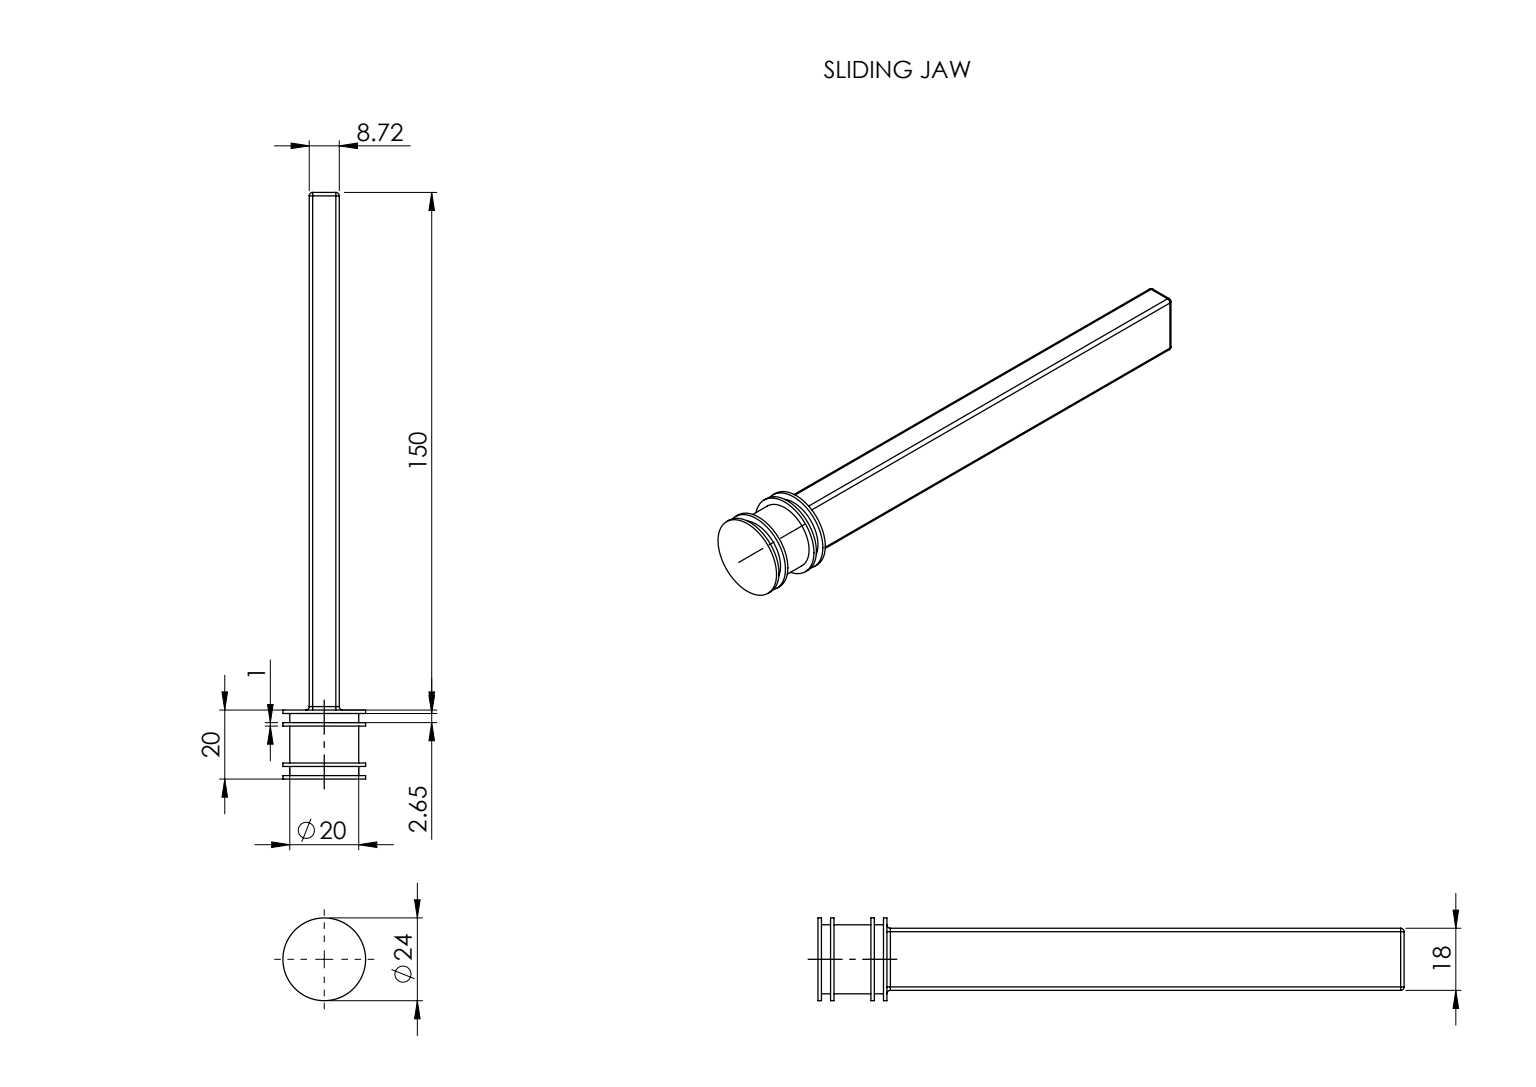
ISO-10303-21;
HEADER;
FILE_DESCRIPTION (('STEP AP214'),
    '1' );
FILE_NAME ('sliding jaw.step',
    '2026-09-29T11:11:29',
    ( '' ),
    ( '' ),
    'SwSTEP 2.0',
    'SolidWorks 2026',
    '' );
FILE_SCHEMA (( 'AUTOMOTIVE_DESIGN' ));
ENDSEC;

DATA;
#4=ORIENTED_EDGE ( 'NONE', *, *, #636, .F. ) ;
#16=DIRECTION ( 'NONE',  ( 0.000000000000000000, 0.000000000000000000, 1.000000000000000000 ) ) ;
#25=DIRECTION ( 'NONE',  ( 1.000000000000000000, 0.000000000000000000, 0.000000000000000000 ) ) ;
#52=CIRCLE ( 'NONE', #6511, 10.00000000000000178 ) ;
#59=CARTESIAN_POINT ( 'NONE',  ( -33.35889894354067309, -7.999999999999996447, -25.00000000000000000 ) ) ;
#82=CARTESIAN_POINT ( 'NONE',  ( -30.00000000000002842, 0.000000000000000000, -44.00000000000000000 ) ) ;
#86=AXIS2_PLACEMENT_3D ( 'NONE', #4207, #8514, #2479 ) ;
#93=SHAPE_DEFINITION_REPRESENTATION ( #6343, #4062 ) ;
#96=CIRCLE ( 'NONE', #1362, 10.00000000000000178 ) ;
#112=VERTEX_POINT ( 'NONE', #3443 ) ;
#118=CARTESIAN_POINT ( 'NONE',  ( -26.64110105645932336, -7.999999999999996447, -23.99999999999999289 ) ) ;
#123=ORIENTED_EDGE ( 'NONE', *, *, #7045, .T. ) ;
#128=CARTESIAN_POINT ( 'NONE',  ( -30.00000000000002842, 0.000000000000000000, -45.00000000000000000 ) ) ;
#157=CIRCLE ( 'NONE', #7186, 11.99999999999979217 ) ;
#159=EDGE_LOOP ( 'NONE', ( #5400, #1966 ) ) ;
#162=CARTESIAN_POINT ( 'NONE',  ( -30.00000000000002842, 0.000000000000000000, -28.65000000000000213 ) ) ;
#164=CARTESIAN_POINT ( 'NONE',  ( -30.00000000000002487, 0.000000000000000000, -25.00000000000000000 ) ) ;
#165=DIRECTION ( 'NONE',  ( -0.000000000000000000, -0.000000000000000000, -1.000000000000000000 ) ) ;
#169=EDGE_LOOP ( 'NONE', ( #3481, #7886, #4, #4040 ) ) ;
#183=CARTESIAN_POINT ( 'NONE',  ( -30.00000000000002842, 10.00000000000000178, -24.00000000000000000 ) ) ;
#194=ORIENTED_EDGE ( 'NONE', *, *, #7448, .F. ) ;
#195=CARTESIAN_POINT ( 'NONE',  ( -33.35889894354067309, -9.999999999999998224, -25.00000000000000000 ) ) ;
#203=FACE_BOUND ( 'NONE', #7034, .T. ) ;
#206=DIRECTION ( 'NONE',  ( -1.000000000000000000, 0.000000000000000000, 0.000000000000000000 ) ) ;
#220=AXIS2_PLACEMENT_3D ( 'NONE', #5235, #7767, #7308 ) ;
#222=CYLINDRICAL_SURFACE ( 'NONE', #8532, 1.000000000000000888 ) ;
#224=LINE ( 'NONE', #3711, #2134 ) ;
#229=CYLINDRICAL_SURFACE ( 'NONE', #3390, 10.00000000000000178 ) ;
#244=PLANE ( 'NONE',  #7417 ) ;
#265=FACE_OUTER_BOUND ( 'NONE', #169, .T. ) ;
#276=CARTESIAN_POINT ( 'NONE',  ( -30.00000000000002487, 0.000000000000000000, -40.35000000000000142 ) ) ;
#280=DIRECTION ( 'NONE',  ( 1.000000000000000000, 0.000000000000000000, 0.000000000000000000 ) ) ;
#300=DIRECTION ( 'NONE',  ( 0.000000000000000000, 0.000000000000000000, 1.000000000000000000 ) ) ;
#303=DIRECTION ( 'NONE',  ( -0.000000000000000000, -0.000000000000000000, -1.000000000000000000 ) ) ;
#315=AXIS2_PLACEMENT_3D ( 'NONE', #2642, #5313, #2599 ) ;
#319=CARTESIAN_POINT ( 'NONE',  ( -26.64110105645932336, -7.999999999999996447, 125.0000000000000000 ) ) ;
#331=SPHERICAL_SURFACE ( 'NONE', #3585, 1.000000000000000000 ) ;
#340=CARTESIAN_POINT ( 'NONE',  ( -26.64110105645932336, 8.000000000000000000, 124.0000000000000000 ) ) ;
#342=DIRECTION ( 'NONE',  ( -1.000000000000000000, 0.000000000000000000, 0.000000000000000000 ) ) ;
#360=EDGE_LOOP ( 'NONE', ( #4155, #3028, #6612 ) ) ;
#381=CARTESIAN_POINT ( 'NONE',  ( -33.35889894354067309, -7.999999999999996447, 124.0000000000000000 ) ) ;
#387=EDGE_LOOP ( 'NONE', ( #8592, #8016, #455, #3412 ) ) ;
#390=PLANE ( 'NONE',  #4662 ) ;
#391=DIRECTION ( 'NONE',  ( 0.000000000000000000, 0.000000000000000000, -1.000000000000000000 ) ) ;
#396=DIRECTION ( 'NONE',  ( 0.000000000000000000, 0.000000000000000000, -1.000000000000000000 ) ) ;
#408=CIRCLE ( 'NONE', #1969, 1.000000000000000888 ) ;
#419=FACE_OUTER_BOUND ( 'NONE', #3879, .T. ) ;
#431=LINE ( 'NONE', #3098, #1438 ) ;
#441=EDGE_CURVE ( 'NONE', #598, #864, #8558, .T. ) ;
#450=ORIENTED_EDGE ( 'NONE', *, *, #3020, .T. ) ;
#455=ORIENTED_EDGE ( 'NONE', *, *, #8086, .F. ) ;
#460=CARTESIAN_POINT ( 'NONE',  ( -30.00000000000002487, 0.000000000000000000, -29.65000000000000213 ) ) ;
#463=ORIENTED_EDGE ( 'NONE', *, *, #2478, .F. ) ;
#466=AXIS2_PLACEMENT_3D ( 'NONE', #6133, #6787, #2038 ) ;
#469=CARTESIAN_POINT ( 'NONE',  ( -26.64110105645932336, 8.000000000000000000, -23.99999999999999289 ) ) ;
#471=CARTESIAN_POINT ( 'NONE',  ( -33.35889894354067309, 8.000000000000000000, 125.0000000000000000 ) ) ;
#477=ORIENTED_EDGE ( 'NONE', *, *, #3290, .F. ) ;
#487=CARTESIAN_POINT ( 'NONE',  ( -18.00000000000023093, 1.469576158976798506E-15, -45.00000000000000000 ) ) ;
#489=TOROIDAL_SURFACE ( 'NONE', #7690, 2.000000000000000000, 1.000000000000000000 ) ;
#506=AXIS2_PLACEMENT_3D ( 'NONE', #7866, #2374, #8526 ) ;
#508=ADVANCED_FACE ( 'NONE', ( #3062, #1146 ), #5739, .F. ) ;
#511=DIRECTION ( 'NONE',  ( 0.000000000000000000, 0.000000000000000000, 1.000000000000000000 ) ) ;
#520=DIRECTION ( 'NONE',  ( 0.000000000000000000, 0.000000000000000000, 1.000000000000000000 ) ) ;
#527=CLOSED_SHELL ( 'NONE', ( #5613, #7239, #5879, #6349, #2268, #2193, #5062, #3908, #2590, #5355, #6240, #6891, #7681, #6961, #3590, #7937, #508, #6501, #1125, #2411, #1851, #6598, #8377, #3918, #1178, #796, #1378, #5792, #2216, #3557, #4936, #1316, #7178, #7893, #8060, #1449, #7304, #1330, #3411, #2383, #6115, #1171, #7572, #8073, #5454, #4555, #3146 ) ) ;
#536=( NAMED_UNIT ( * ) SI_UNIT ( $, .STERADIAN. ) SOLID_ANGLE_UNIT ( ) );
#537=ORIENTED_EDGE ( 'NONE', *, *, #6250, .F. ) ;
#538=DIRECTION ( 'NONE',  ( 0.000000000000000000, 0.000000000000000000, -1.000000000000000000 ) ) ;
#563=CARTESIAN_POINT ( 'NONE',  ( -42.00000000000002132, 0.000000000000000000, -29.65000000000000213 ) ) ;
#572=PLANE ( 'NONE',  #1496 ) ;
#580=VERTEX_POINT ( 'NONE', #7145 ) ;
#586=ORIENTED_EDGE ( 'NONE', *, *, #2638, .T. ) ;
#590=( LENGTH_UNIT ( ) NAMED_UNIT ( * ) SI_UNIT ( .MILLI., .METRE. ) );
#595=EDGE_LOOP ( 'NONE', ( #4745, #2458, #2730, #1335 ) ) ;
#598=VERTEX_POINT ( 'NONE', #8559 ) ;
#615=CARTESIAN_POINT ( 'NONE',  ( -26.64110105645932336, 9.000000000000001776, 125.0000000000000000 ) ) ;
#618=LINE ( 'NONE', #2581, #6843 ) ;
#627=AXIS2_PLACEMENT_3D ( 'NONE', #1489, #300, #3700 ) ;
#636=EDGE_CURVE ( 'NONE', #5681, #7609, #5596, .T. ) ;
#644=DIRECTION ( 'NONE',  ( 1.000000000000000000, 0.000000000000000000, 0.000000000000000000 ) ) ;
#653=AXIS2_PLACEMENT_3D ( 'NONE', #4860, #1588, #6305 ) ;
#658=CARTESIAN_POINT ( 'NONE',  ( -17.99999999999998579, 1.469576158976828483E-15, -29.65000000000000213 ) ) ;
#659=DIRECTION ( 'NONE',  ( -0.000000000000000000, -0.000000000000000000, -1.000000000000000000 ) ) ;
#661=ORIENTED_EDGE ( 'NONE', *, *, #5691, .T. ) ;
#673=ORIENTED_EDGE ( 'NONE', *, *, #4128, .F. ) ;
#697=DIRECTION ( 'NONE',  ( -1.000000000000000000, 0.000000000000000000, 0.000000000000000000 ) ) ;
#706=AXIS2_PLACEMENT_3D ( 'NONE', #5991, #697, #8325 ) ;
#714=CARTESIAN_POINT ( 'NONE',  ( -40.00000000000002842, 1.224646799147353059E-15, -40.35000000000000142 ) ) ;
#725=ORIENTED_EDGE ( 'NONE', *, *, #7163, .T. ) ;
#731=DIRECTION ( 'NONE',  ( 0.000000000000000000, -1.000000000000000000, 0.000000000000000000 ) ) ;
#733=ORIENTED_EDGE ( 'NONE', *, *, #8138, .T. ) ;
#771=EDGE_CURVE ( 'NONE', #772, #7794, #6358, .T. ) ;
#772=VERTEX_POINT ( 'NONE', #3873 ) ;
#774=CARTESIAN_POINT ( 'NONE',  ( -26.64110105645932336, -9.999999999999998224, -24.00000000000000000 ) ) ;
#776=DIRECTION ( 'NONE',  ( -1.000000000000000000, 0.000000000000000000, 0.000000000000000000 ) ) ;
#796=ADVANCED_FACE ( 'NONE', ( #3827 ), #6507, .T. ) ;
#806=DIRECTION ( 'NONE',  ( 1.000000000000000000, 0.000000000000000000, -0.000000000000000000 ) ) ;
#812=ORIENTED_EDGE ( 'NONE', *, *, #2573, .F. ) ;
#818=EDGE_CURVE ( 'NONE', #7794, #1195, #3435, .T. ) ;
#822=CARTESIAN_POINT ( 'NONE',  ( -30.00000000000002842, 0.000000000000000000, -40.35000000000000142 ) ) ;
#824=ORIENTED_EDGE ( 'NONE', *, *, #8649, .T. ) ;
#830=CARTESIAN_POINT ( 'NONE',  ( -33.35889894354067309, -7.999999999999996447, -23.99999999999999289 ) ) ;
#849=CIRCLE ( 'NONE', #6478, 10.00000000000000178 ) ;
#852=PLANE ( 'NONE',  #1788 ) ;
#853=ORIENTED_EDGE ( 'NONE', *, *, #886, .F. ) ;
#859=CARTESIAN_POINT ( 'NONE',  ( -20.00000000000002487, 0.000000000000000000, -41.34999999999999432 ) ) ;
#860=DIRECTION ( 'NONE',  ( 0.000000000000000000, 0.000000000000000000, 1.000000000000000000 ) ) ;
#862=CARTESIAN_POINT ( 'NONE',  ( -30.00000000000002487, 0.000000000000000000, -29.65000000000000213 ) ) ;
#864=VERTEX_POINT ( 'NONE', #1218 ) ;
#881=AXIS2_PLACEMENT_3D ( 'NONE', #1764, #2549, #8503 ) ;
#886=EDGE_CURVE ( 'NONE', #2202, #3619, #5942, .T. ) ;
#888=AXIS2_PLACEMENT_3D ( 'NONE', #1840, #2501, #538 ) ;
#893=EDGE_CURVE ( 'NONE', #4571, #5715, #1301, .T. ) ;
#903=VECTOR ( 'NONE', #7606, 1000.000000000000000 ) ;
#909=LINE ( 'NONE', #6766, #903 ) ;
#931=CARTESIAN_POINT ( 'NONE',  ( -40.00000000000002842, 1.224646799147353059E-15, -26.00000000000000355 ) ) ;
#932=TOROIDAL_SURFACE ( 'NONE', #1494, 2.000000000000000000, 1.000000000000000000 ) ;
#946=AXIS2_PLACEMENT_3D ( 'NONE', #774, #5439, #860 ) ;
#950=CARTESIAN_POINT ( 'NONE',  ( -26.64110105645932336, -8.999999999999998224, -24.00000000000000000 ) ) ;
#952=DIRECTION ( 'NONE',  ( 0.000000000000000000, 0.000000000000000000, 1.000000000000000000 ) ) ;
#955=ORIENTED_EDGE ( 'NONE', *, *, #6438, .T. ) ;
#959=EDGE_LOOP ( 'NONE', ( #4655, #2762 ) ) ;
#964=CARTESIAN_POINT ( 'NONE',  ( -34.35889894354067309, -8.999999999999998224, -24.00000000000000000 ) ) ;
#973=DIRECTION ( 'NONE',  ( 0.000000000000000000, 0.000000000000000000, 1.000000000000000000 ) ) ;
#989=CARTESIAN_POINT ( 'NONE',  ( -26.64110105645932336, 9.000000000000001776, -24.00000000000000000 ) ) ;
#998=CIRCLE ( 'NONE', #4381, 1.000000000000000888 ) ;
#999=VERTEX_POINT ( 'NONE', #7967 ) ;
#1007=EDGE_CURVE ( 'NONE', #4525, #7472, #6705, .T. ) ;
#1009=VERTEX_POINT ( 'NONE', #4000 ) ;
#1012=ORIENTED_EDGE ( 'NONE', *, *, #6438, .F. ) ;
#1019=DIRECTION ( 'NONE',  ( -0.000000000000000000, -0.000000000000000000, -1.000000000000000000 ) ) ;
#1021=CIRCLE ( 'NONE', #5949, 1.000000000000000888 ) ;
#1039=CARTESIAN_POINT ( 'NONE',  ( -35.35889894354067309, 0.000000000000000000, -24.00000000000000000 ) ) ;
#1044=CIRCLE ( 'NONE', #6810, 10.00000000000000178 ) ;
#1046=VERTEX_POINT ( 'NONE', #950 ) ;
#1059=DIRECTION ( 'NONE',  ( 0.000000000000000000, 0.000000000000000000, -1.000000000000000000 ) ) ;
#1065=CARTESIAN_POINT ( 'NONE',  ( -33.35889894354067309, 10.00000000000000178, -25.00000000000000000 ) ) ;
#1072=VERTEX_POINT ( 'NONE', #3758 ) ;
#1083=EDGE_LOOP ( 'NONE', ( #3654, #4068, #5069, #1575 ) ) ;
#1092=CARTESIAN_POINT ( 'NONE',  ( -25.64110105645932336, 8.000000000000000000, 125.0000000000000000 ) ) ;
#1094=FACE_OUTER_BOUND ( 'NONE', #2864, .T. ) ;
#1112=ORIENTED_EDGE ( 'NONE', *, *, #3664, .T. ) ;
#1117=CARTESIAN_POINT ( 'NONE',  ( -42.00000000000002132, 0.000000000000000000, -28.65000000000000213 ) ) ;
#1125=ADVANCED_FACE ( 'NONE', ( #203, #4882 ), #244, .F. ) ;
#1146=FACE_OUTER_BOUND ( 'NONE', #3517, .T. ) ;
#1148=EDGE_CURVE ( 'NONE', #1263, #1046, #2502, .T. ) ;
#1157=EDGE_CURVE ( 'NONE', #4571, #3127, #4461, .T. ) ;
#1164=DIRECTION ( 'NONE',  ( -1.000000000000000000, 0.000000000000000000, 0.000000000000000000 ) ) ;
#1171=ADVANCED_FACE ( 'NONE', ( #4922 ), #8239, .T. ) ;
#1172=CIRCLE ( 'NONE', #6516, 10.00000000000000178 ) ;
#1177=CARTESIAN_POINT ( 'NONE',  ( -42.00000000000006395, 0.000000000000000000, -29.65000000000000213 ) ) ;
#1178=ADVANCED_FACE ( 'NONE', ( #5574, #8282 ), #2243, .F. ) ;
#1182=VECTOR ( 'NONE', #7954, 1000.000000000000000 ) ;
#1183=ORIENTED_EDGE ( 'NONE', *, *, #2611, .F. ) ;
#1189=EDGE_CURVE ( 'NONE', #5443, #1675, #4966, .T. ) ;
#1192=DIRECTION ( 'NONE',  ( -0.000000000000000000, 1.000000000000000000, 0.000000000000000000 ) ) ;
#1195=VERTEX_POINT ( 'NONE', #2111 ) ;
#1208=AXIS2_PLACEMENT_3D ( 'NONE', #2158, #8155, #3438 ) ;
#1215=ORIENTED_EDGE ( 'NONE', *, *, #8346, .F. ) ;
#1218=CARTESIAN_POINT ( 'NONE',  ( -24.64110105645932336, 8.000000000000000000, -25.00000000000000000 ) ) ;
#1219=FACE_OUTER_BOUND ( 'NONE', #2950, .T. ) ;
#1226=CYLINDRICAL_SURFACE ( 'NONE', #220, 12.00000000000000000 ) ;
#1235=CARTESIAN_POINT ( 'NONE',  ( -24.64110105645932336, -8.999999999999998224, -25.00000000000000000 ) ) ;
#1239=DIRECTION ( 'NONE',  ( 0.000000000000000000, 1.000000000000000000, -0.000000000000000000 ) ) ;
#1243=DIRECTION ( 'NONE',  ( -0.000000000000000000, -0.000000000000000000, -1.000000000000000000 ) ) ;
#1254=ORIENTED_EDGE ( 'NONE', *, *, #636, .T. ) ;
#1263=VERTEX_POINT ( 'NONE', #6917 ) ;
#1265=EDGE_CURVE ( 'NONE', #2617, #8337, #8133, .T. ) ;
#1275=DIRECTION ( 'NONE',  ( -1.000000000000000000, 0.000000000000000000, 0.000000000000000000 ) ) ;
#1279=CARTESIAN_POINT ( 'NONE',  ( -24.64110105645932336, 0.000000000000000000, -24.00000000000000000 ) ) ;
#1287=LINE ( 'NONE', #5256, #1182 ) ;
#1300=( NAMED_UNIT ( * ) PLANE_ANGLE_UNIT ( ) SI_UNIT ( $, .RADIAN. ) );
#1301=LINE ( 'NONE', #5396, #2999 ) ;
#1316=ADVANCED_FACE ( 'NONE', ( #2172 ), #222, .F. ) ;
#1321=CARTESIAN_POINT ( 'NONE',  ( -34.35889894354067309, 8.000000000000000000, 124.0000000000000000 ) ) ;
#1327=CARTESIAN_POINT ( 'NONE',  ( -26.64110105645932336, -7.999999999999996447, 124.0000000000000000 ) ) ;
#1330=ADVANCED_FACE ( 'NONE', ( #265 ), #489, .F. ) ;
#1332=CYLINDRICAL_SURFACE ( 'NONE', #3852, 1.000000000000000888 ) ;
#1334=( NAMED_UNIT ( * ) PLANE_ANGLE_UNIT ( ) SI_UNIT ( $, .RADIAN. ) );
#1335=ORIENTED_EDGE ( 'NONE', *, *, #5477, .T. ) ;
#1345=DIRECTION ( 'NONE',  ( -1.000000000000000000, 0.000000000000000000, 0.000000000000000000 ) ) ;
#1348=CARTESIAN_POINT ( 'NONE',  ( -30.00000000000002842, 0.000000000000000000, -45.00000000000000000 ) ) ;
#1362=AXIS2_PLACEMENT_3D ( 'NONE', #5707, #8409, #1701 ) ;
#1378=ADVANCED_FACE ( 'NONE', ( #6728 ), #5228, .F. ) ;
#1388=ORIENTED_EDGE ( 'NONE', *, *, #8346, .T. ) ;
#1389=EDGE_LOOP ( 'NONE', ( #2321, #2903 ) ) ;
#1391=CARTESIAN_POINT ( 'NONE',  ( -25.64110105645932336, 8.000000000000000000, 124.0000000000000000 ) ) ;
#1394=DIRECTION ( 'NONE',  ( 0.000000000000000000, 0.000000000000000000, -1.000000000000000000 ) ) ;
#1395=CARTESIAN_POINT ( 'NONE',  ( -35.35889894354067309, 8.000000000000000000, -24.00000000000000000 ) ) ;
#1427=EDGE_LOOP ( 'NONE', ( #3891, #3996 ) ) ;
#1438=VECTOR ( 'NONE', #5779, 1000.000000000000000 ) ;
#1443=ORIENTED_EDGE ( 'NONE', *, *, #6341, .T. ) ;
#1449=ADVANCED_FACE ( 'NONE', ( #8285 ), #2862, .T. ) ;
#1464=EDGE_CURVE ( 'NONE', #8429, #5042, #3565, .T. ) ;
#1472=ORIENTED_EDGE ( 'NONE', *, *, #6300, .T. ) ;
#1481=CARTESIAN_POINT ( 'NONE',  ( -34.35889894354067309, -7.999999999999996447, 125.0000000000000000 ) ) ;
#1486=EDGE_LOOP ( 'NONE', ( #3350, #2470 ) ) ;
#1489=CARTESIAN_POINT ( 'NONE',  ( -30.00000000000002842, 0.000000000000000000, -45.00000000000000000 ) ) ;
#1494=AXIS2_PLACEMENT_3D ( 'NONE', #7551, #1514, #280 ) ;
#1496=AXIS2_PLACEMENT_3D ( 'NONE', #3239, #2709, #6749 ) ;
#1503=AXIS2_PLACEMENT_3D ( 'NONE', #3408, #7897, #1275 ) ;
#1508=AXIS2_PLACEMENT_3D ( 'NONE', #5913, #2660, #8687 ) ;
#1514=DIRECTION ( 'NONE',  ( 0.000000000000000000, 0.000000000000000000, 1.000000000000000000 ) ) ;
#1519=ORIENTED_EDGE ( 'NONE', *, *, #1781, .F. ) ;
#1522=DIRECTION ( 'NONE',  ( -1.000000000000000000, 0.000000000000000000, 0.000000000000000000 ) ) ;
#1537=ORIENTED_EDGE ( 'NONE', *, *, #4588, .T. ) ;
#1545=CARTESIAN_POINT ( 'NONE',  ( -30.00000000000002842, 0.000000000000000000, -41.34999999999999432 ) ) ;
#1554=VECTOR ( 'NONE', #2289, 1000.000000000000000 ) ;
#1558=ORIENTED_EDGE ( 'NONE', *, *, #7155, .F. ) ;
#1567=LINE ( 'NONE', #7478, #7656 ) ;
#1575=ORIENTED_EDGE ( 'NONE', *, *, #6921, .F. ) ;
#1581=DIRECTION ( 'NONE',  ( 0.000000000000000000, 0.000000000000000000, 1.000000000000000000 ) ) ;
#1583=ORIENTED_EDGE ( 'NONE', *, *, #2646, .F. ) ;
#1587=AXIS2_PLACEMENT_3D ( 'NONE', #2835, #3455, #8171 ) ;
#1588=DIRECTION ( 'NONE',  ( 0.000000000000000000, -0.000000000000000000, 1.000000000000000000 ) ) ;
#1590=CARTESIAN_POINT ( 'NONE',  ( -33.35889894354067309, -9.999999999999998224, -24.00000000000000000 ) ) ;
#1604=ORIENTED_EDGE ( 'NONE', *, *, #8180, .F. ) ;
#1608=AXIS2_PLACEMENT_3D ( 'NONE', #2572, #5245, #8717 ) ;
#1609=EDGE_CURVE ( 'NONE', #3466, #3121, #6430, .T. ) ;
#1612=CARTESIAN_POINT ( 'NONE',  ( -30.00000000000023093, 0.000000000000000000, -44.00000000000000000 ) ) ;
#1616=DIRECTION ( 'NONE',  ( 0.000000000000000000, 0.000000000000000000, 1.000000000000000000 ) ) ;
#1642=EDGE_CURVE ( 'NONE', #3619, #6952, #5026, .T. ) ;
#1647=CIRCLE ( 'NONE', #6298, 1.000000000000000888 ) ;
#1654=VECTOR ( 'NONE', #2362, 1000.000000000000000 ) ;
#1660=CARTESIAN_POINT ( 'NONE',  ( -26.64110105645932336, -7.999999999999996447, 124.0000000000000000 ) ) ;
#1663=VERTEX_POINT ( 'NONE', #859 ) ;
#1675=VERTEX_POINT ( 'NONE', #6365 ) ;
#1679=DIRECTION ( 'NONE',  ( 0.000000000000000000, 0.000000000000000000, 1.000000000000000000 ) ) ;
#1681=LINE ( 'NONE', #6437, #4511 ) ;
#1690=CARTESIAN_POINT ( 'NONE',  ( -41.99999999999981526, 0.000000000000000000, -44.00000000000000000 ) ) ;
#1694=ORIENTED_EDGE ( 'NONE', *, *, #3020, .F. ) ;
#1701=DIRECTION ( 'NONE',  ( 1.000000000000000000, 0.000000000000000000, 0.000000000000000000 ) ) ;
#1707=DIRECTION ( 'NONE',  ( 0.000000000000000000, 0.000000000000000000, 1.000000000000000000 ) ) ;
#1719=DIRECTION ( 'NONE',  ( -1.000000000000000000, 0.000000000000000000, 0.000000000000000000 ) ) ;
#1721=ORIENTED_EDGE ( 'NONE', *, *, #1642, .T. ) ;
#1723=EDGE_CURVE ( 'NONE', #1046, #5443, #2412, .T. ) ;
#1731=FACE_BOUND ( 'NONE', #6833, .T. ) ;
#1732=DIRECTION ( 'NONE',  ( -1.000000000000000000, 0.000000000000000000, 0.000000000000000000 ) ) ;
#1735=VECTOR ( 'NONE', #3213, 1000.000000000000000 ) ;
#1744=VECTOR ( 'NONE', #7293, 1000.000000000000000 ) ;
#1757=ORIENTED_EDGE ( 'NONE', *, *, #818, .F. ) ;
#1764=CARTESIAN_POINT ( 'NONE',  ( -30.00000000000002487, 0.000000000000000000, -41.35000000000000142 ) ) ;
#1775=DIRECTION ( 'NONE',  ( 1.000000000000000000, 0.000000000000000000, -0.000000000000000000 ) ) ;
#1776=AXIS2_PLACEMENT_3D ( 'NONE', #4486, #5186, #6424 ) ;
#1779=CARTESIAN_POINT ( 'NONE',  ( -30.00000000000002487, 0.000000000000000000, -28.65000000000000213 ) ) ;
#1781=EDGE_CURVE ( 'NONE', #5443, #3221, #5287, .T. ) ;
#1782=DIRECTION ( 'NONE',  ( 1.000000000000000000, 0.000000000000000000, 0.000000000000000000 ) ) ;
#1788=AXIS2_PLACEMENT_3D ( 'NONE', #4252, #2234, #6318 ) ;
#1793=FACE_OUTER_BOUND ( 'NONE', #1083, .T. ) ;
#1801=ORIENTED_EDGE ( 'NONE', *, *, #8649, .F. ) ;
#1805=CARTESIAN_POINT ( 'NONE',  ( -40.00000000000002842, 1.224646799147353256E-15, -45.00000000000000000 ) ) ;
#1822=EDGE_CURVE ( 'NONE', #3764, #5405, #618, .T. ) ;
#1830=CARTESIAN_POINT ( 'NONE',  ( -34.35889894354067309, 9.000000000000001776, 125.0000000000000000 ) ) ;
#1840=CARTESIAN_POINT ( 'NONE',  ( -33.35889894354067309, -8.999999999999998224, 124.0000000000000000 ) ) ;
#1848=LINE ( 'NONE', #3787, #7361 ) ;
#1851=ADVANCED_FACE ( 'NONE', ( #7906, #1872 ), #572, .F. ) ;
#1861=DIRECTION ( 'NONE',  ( -0.000000000000000000, -1.000000000000000000, -0.000000000000000000 ) ) ;
#1872=FACE_OUTER_BOUND ( 'NONE', #3259, .T. ) ;
#1877=DIRECTION ( 'NONE',  ( 0.000000000000000000, 0.000000000000000000, 1.000000000000000000 ) ) ;
#1878=CIRCLE ( 'NONE', #881, 11.99999999999983302 ) ;
#1893=AXIS2_PLACEMENT_3D ( 'NONE', #164, #2861, #5536 ) ;
#1896=ORIENTED_EDGE ( 'NONE', *, *, #8180, .T. ) ;
#1901=CARTESIAN_POINT ( 'NONE',  ( -20.00000000000002487, 0.000000000000000000, -40.35000000000000142 ) ) ;
#1905=DIRECTION ( 'NONE',  ( -0.000000000000000000, -0.000000000000000000, -1.000000000000000000 ) ) ;
#1925=VERTEX_POINT ( 'NONE', #2532 ) ;
#1926=AXIS2_PLACEMENT_3D ( 'NONE', #4885, #165, #206 ) ;
#1930=CARTESIAN_POINT ( 'NONE',  ( -30.00000000000002487, 0.000000000000000000, -45.00000000000000000 ) ) ;
#1934=ORIENTED_EDGE ( 'NONE', *, *, #3311, .T. ) ;
#1935=AXIS2_PLACEMENT_3D ( 'NONE', #8305, #6923, #2178 ) ;
#1961=DIRECTION ( 'NONE',  ( -1.000000000000000000, -0.000000000000000000, -0.000000000000000000 ) ) ;
#1965=ORIENTED_EDGE ( 'NONE', *, *, #7880, .T. ) ;
#1966=ORIENTED_EDGE ( 'NONE', *, *, #7163, .F. ) ;
#1969=AXIS2_PLACEMENT_3D ( 'NONE', #6964, #3095, #5117 ) ;
#1978=AXIS2_PLACEMENT_3D ( 'NONE', #4643, #7423, #7331 ) ;
#1982=CIRCLE ( 'NONE', #5347, 1.000000000000000888 ) ;
#1987=( GEOMETRIC_REPRESENTATION_CONTEXT ( 3 ) GLOBAL_UNCERTAINTY_ASSIGNED_CONTEXT ( ( #3854 ) ) GLOBAL_UNIT_ASSIGNED_CONTEXT ( ( #8044, #1334, #536 ) ) REPRESENTATION_CONTEXT ( 'NONE', 'WORKASPACE' ) );
#1991=FACE_OUTER_BOUND ( 'NONE', #3804, .T. ) ;
#1994=ORIENTED_EDGE ( 'NONE', *, *, #7332, .T. ) ;
#2003=PLANE ( 'NONE',  #4144 ) ;
#2005=( NAMED_UNIT ( * ) PLANE_ANGLE_UNIT ( ) SI_UNIT ( $, .RADIAN. ) );
#2018=DIRECTION ( 'NONE',  ( 1.000000000000000000, -0.000000000000000000, -0.000000000000000000 ) ) ;
#2034=CIRCLE ( 'NONE', #1893, 12.00000000000004263 ) ;
#2038=DIRECTION ( 'NONE',  ( 1.000000000000000000, 0.000000000000000000, 0.000000000000000000 ) ) ;
#2041=LINE ( 'NONE', #615, #2787 ) ;
#2053=DIRECTION ( 'NONE',  ( 1.000000000000000000, 0.000000000000000000, 0.000000000000000000 ) ) ;
#2085=DIRECTION ( 'NONE',  ( -1.000000000000000000, -0.000000000000000000, 0.000000000000000000 ) ) ;
#2101=DIRECTION ( 'NONE',  ( 0.000000000000000000, 0.000000000000000000, 1.000000000000000000 ) ) ;
#2110=FILL_AREA_STYLE_COLOUR ( '', #8071 ) ;
#2111=CARTESIAN_POINT ( 'NONE',  ( -26.64110105645932336, -7.999999999999996447, 125.0000000000000000 ) ) ;
#2134=VECTOR ( 'NONE', #1059, 1000.000000000000000 ) ;
#2141=FACE_BOUND ( 'NONE', #3876, .T. ) ;
#2145=ORIENTED_EDGE ( 'NONE', *, *, #7045, .F. ) ;
#2150=VERTEX_POINT ( 'NONE', #3923 ) ;
#2154=VECTOR ( 'NONE', #1019, 1000.000000000000000 ) ;
#2155=DIRECTION ( 'NONE',  ( 1.000000000000000000, 0.000000000000000000, -0.000000000000000000 ) ) ;
#2157=DIRECTION ( 'NONE',  ( 0.000000000000000000, 0.000000000000000000, 1.000000000000000000 ) ) ;
#2158=CARTESIAN_POINT ( 'NONE',  ( -26.64110105645932336, -8.999999999999998224, 124.0000000000000000 ) ) ;
#2159=ORIENTED_EDGE ( 'NONE', *, *, #8544, .F. ) ;
#2162=CIRCLE ( 'NONE', #4410, 10.00000000000000178 ) ;
#2163=MECHANICAL_DESIGN_GEOMETRIC_PRESENTATION_REPRESENTATION('',(#3433),#6648);
#2164=ORIENTED_EDGE ( 'NONE', *, *, #1723, .T. ) ;
#2168=FACE_OUTER_BOUND ( 'NONE', #3180, .T. ) ;
#2172=FACE_OUTER_BOUND ( 'NONE', #387, .T. ) ;
#2175=VECTOR ( 'NONE', #6200, 1000.000000000000000 ) ;
#2177=VERTEX_POINT ( 'NONE', #4421 ) ;
#2178=DIRECTION ( 'NONE',  ( -1.000000000000000000, 0.000000000000000000, 0.000000000000000000 ) ) ;
#2193=ADVANCED_FACE ( 'NONE', ( #5078 ), #6441, .T. ) ;
#2196=CARTESIAN_POINT ( 'NONE',  ( -30.00000000000002842, 0.000000000000000000, -41.34999999999999432 ) ) ;
#2197=DIRECTION ( 'NONE',  ( 0.000000000000000000, 0.000000000000000000, -1.000000000000000000 ) ) ;
#2202=VERTEX_POINT ( 'NONE', #1065 ) ;
#2216=ADVANCED_FACE ( 'NONE', ( #6311 ), #4586, .F. ) ;
#2228=AXIS2_PLACEMENT_3D ( 'NONE', #7409, #4591, #5955 ) ;
#2234=DIRECTION ( 'NONE',  ( 0.000000000000000000, 0.000000000000000000, 1.000000000000000000 ) ) ;
#2243=PLANE ( 'NONE',  #6295 ) ;
#2245=CARTESIAN_POINT ( 'NONE',  ( -26.64110105645932336, -7.999999999999996447, 124.0000000000000000 ) ) ;
#2246=DIRECTION ( 'NONE',  ( 0.000000000000000000, 0.000000000000000000, 1.000000000000000000 ) ) ;
#2247=EDGE_LOOP ( 'NONE', ( #8564, #6360 ) ) ;
#2268=ADVANCED_FACE ( 'NONE', ( #3672 ), #1226, .T. ) ;
#2278=ORIENTED_EDGE ( 'NONE', *, *, #8254, .F. ) ;
#2289=DIRECTION ( 'NONE',  ( -1.000000000000000000, -0.000000000000000000, -0.000000000000000000 ) ) ;
#2300=DIRECTION ( 'NONE',  ( 1.000000000000000000, 0.000000000000000000, 0.000000000000000000 ) ) ;
#2307=CIRCLE ( 'NONE', #7360, 1.000000000000000888 ) ;
#2311=DIRECTION ( 'NONE',  ( -0.000000000000000000, -0.000000000000000000, -1.000000000000000000 ) ) ;
#2321=ORIENTED_EDGE ( 'NONE', *, *, #1609, .T. ) ;
#2322=CARTESIAN_POINT ( 'NONE',  ( -33.35889894354067309, 8.000000000000000000, 124.0000000000000000 ) ) ;
#2345=PRODUCT ( 'sliding jaw', 'sliding jaw', '', ( #6134 ) ) ;
#2352=LINE ( 'NONE', #4945, #3676 ) ;
#2362=DIRECTION ( 'NONE',  ( -1.000000000000000000, 0.000000000000000000, 0.000000000000000000 ) ) ;
#2364=CIRCLE ( 'NONE', #506, 10.00000000000000178 ) ;
#2367=ORIENTED_EDGE ( 'NONE', *, *, #8442, .F. ) ;
#2374=DIRECTION ( 'NONE',  ( -0.000000000000000000, -0.000000000000000000, -1.000000000000000000 ) ) ;
#2383=ADVANCED_FACE ( 'NONE', ( #4932 ), #2958, .T. ) ;
#2384=ORIENTED_EDGE ( 'NONE', *, *, #8442, .T. ) ;
#2396=CARTESIAN_POINT ( 'NONE',  ( -33.35889894354067309, -7.999999999999996447, 124.0000000000000000 ) ) ;
#2399=DIRECTION ( 'NONE',  ( 0.000000000000000000, 0.000000000000000000, -1.000000000000000000 ) ) ;
#2406=ORIENTED_EDGE ( 'NONE', *, *, #3223, .F. ) ;
#2410=CIRCLE ( 'NONE', #5487, 1.000000000000000888 ) ;
#2411=ADVANCED_FACE ( 'NONE', ( #3614 ), #7529, .T. ) ;
#2412=LINE ( 'NONE', #3809, #5727 ) ;
#2425=CARTESIAN_POINT ( 'NONE',  ( -33.35889894354067309, 9.000000000000001776, 125.0000000000000000 ) ) ;
#2427=STYLED_ITEM ( 'NONE', ( #6012 ), #2772 ) ;
#2433=ORIENTED_EDGE ( 'NONE', *, *, #818, .T. ) ;
#2436=AXIS2_PLACEMENT_3D ( 'NONE', #128, #1581, #7531 ) ;
#2458=ORIENTED_EDGE ( 'NONE', *, *, #6769, .T. ) ;
#2465=CARTESIAN_POINT ( 'NONE',  ( -30.00000000000002487, 0.000000000000000000, -29.65000000000000213 ) ) ;
#2470=ORIENTED_EDGE ( 'NONE', *, *, #2478, .T. ) ;
#2478=EDGE_CURVE ( 'NONE', #7472, #4525, #7823, .T. ) ;
#2479=DIRECTION ( 'NONE',  ( -1.000000000000000000, 0.000000000000000000, 0.000000000000000000 ) ) ;
#2484=LINE ( 'NONE', #5164, #6164 ) ;
#2497=DIRECTION ( 'NONE',  ( -0.000000000000000000, -0.000000000000000000, -1.000000000000000000 ) ) ;
#2501=DIRECTION ( 'NONE',  ( 0.000000000000000000, -1.000000000000000000, 0.000000000000000000 ) ) ;
#2502=CIRCLE ( 'NONE', #946, 1.000000000000000888 ) ;
#2505=AXIS2_PLACEMENT_3D ( 'NONE', #5133, #5794, #4433 ) ;
#2526=EDGE_CURVE ( 'NONE', #5895, #3379, #1878, .T. ) ;
#2528=ORIENTED_EDGE ( 'NONE', *, *, #7148, .F. ) ;
#2532=CARTESIAN_POINT ( 'NONE',  ( -20.00000000000002487, 0.000000000000000000, -44.00000000000000000 ) ) ;
#2537=CARTESIAN_POINT ( 'NONE',  ( -33.35889894354067309, -8.999999999999998224, -24.00000000000000000 ) ) ;
#2549=DIRECTION ( 'NONE',  ( -0.000000000000000000, -0.000000000000000000, -1.000000000000000000 ) ) ;
#2554=AXIS2_PLACEMENT_3D ( 'NONE', #7787, #1707, #3692 ) ;
#2565=EDGE_CURVE ( 'NONE', #1072, #5184, #3012, .T. ) ;
#2567=AXIS2_PLACEMENT_3D ( 'NONE', #381, #8504, #8465 ) ;
#2572=CARTESIAN_POINT ( 'NONE',  ( -30.00000000000002842, 0.000000000000000000, -40.35000000000000142 ) ) ;
#2573=EDGE_CURVE ( 'NONE', #5405, #3069, #1848, .T. ) ;
#2581=CARTESIAN_POINT ( 'NONE',  ( -26.64110105645932336, 9.000000000000001776, 125.0000000000000000 ) ) ;
#2588=ORIENTED_EDGE ( 'NONE', *, *, #1822, .F. ) ;
#2590=ADVANCED_FACE ( 'NONE', ( #8463 ), #6464, .T. ) ;
#2599=DIRECTION ( 'NONE',  ( 0.000000000000000000, -0.000000000000000000, -1.000000000000000000 ) ) ;
#2601=CIRCLE ( 'NONE', #8645, 1.000000000000000888 ) ;
#2611=EDGE_CURVE ( 'NONE', #4408, #112, #8629, .T. ) ;
#2617=VERTEX_POINT ( 'NONE', #3741 ) ;
#2626=FACE_OUTER_BOUND ( 'NONE', #7846, .T. ) ;
#2634=CIRCLE ( 'NONE', #86, 12.00000000000004263 ) ;
#2638=EDGE_CURVE ( 'NONE', #7971, #3466, #6506, .T. ) ;
#2642=CARTESIAN_POINT ( 'NONE',  ( -34.35889894354067309, -8.999999999999998224, 125.0000000000000000 ) ) ;
#2646=EDGE_CURVE ( 'NONE', #3069, #2617, #7256, .T. ) ;
#2649=AXIS2_PLACEMENT_3D ( 'NONE', #7988, #1192, #4020 ) ;
#2660=DIRECTION ( 'NONE',  ( -0.000000000000000000, -0.000000000000000000, -1.000000000000000000 ) ) ;
#2671=LINE ( 'NONE', #6538, #5391 ) ;
#2674=CARTESIAN_POINT ( 'NONE',  ( -26.64110105645932336, -7.999999999999996447, -25.00000000000000000 ) ) ;
#2699=EDGE_CURVE ( 'NONE', #598, #2752, #7129, .T. ) ;
#2709=DIRECTION ( 'NONE',  ( -0.000000000000000000, 0.000000000000000000, -1.000000000000000000 ) ) ;
#2710=CARTESIAN_POINT ( 'NONE',  ( -30.00000000000002487, 0.000000000000000000, -29.65000000000000213 ) ) ;
#2715=CIRCLE ( 'NONE', #7630, 12.00000000000000000 ) ;
#2721=VERTEX_POINT ( 'NONE', #6109 ) ;
#2725=AXIS2_PLACEMENT_3D ( 'NONE', #2465, #3174, #5147 ) ;
#2730=ORIENTED_EDGE ( 'NONE', *, *, #893, .T. ) ;
#2750=DIRECTION ( 'NONE',  ( -0.000000000000000000, -0.000000000000000000, -1.000000000000000000 ) ) ;
#2752=VERTEX_POINT ( 'NONE', #1391 ) ;
#2757=DIRECTION ( 'NONE',  ( 0.000000000000000000, 0.000000000000000000, 1.000000000000000000 ) ) ;
#2762=ORIENTED_EDGE ( 'NONE', *, *, #7138, .F. ) ;
#2768=ORIENTED_EDGE ( 'NONE', *, *, #7411, .F. ) ;
#2772=ADVANCED_BREP_SHAPE_REPRESENTATION ( '', ( #2885, #2554 ), #1987 ) ;
#2779=AXIS2_PLACEMENT_3D ( 'NONE', #8663, #1961, #5343 ) ;
#2787=VECTOR ( 'NONE', #5332, 1000.000000000000000 ) ;
#2789=DIRECTION ( 'NONE',  ( 0.000000000000000000, 0.000000000000000000, 1.000000000000000000 ) ) ;
#2791=CIRCLE ( 'NONE', #3909, 1.000000000000000888 ) ;
#2795=ORIENTED_EDGE ( 'NONE', *, *, #2611, .T. ) ;
#2804=ORIENTED_EDGE ( 'NONE', *, *, #8524, .T. ) ;
#2806=ORIENTED_EDGE ( 'NONE', *, *, #4721, .T. ) ;
#2811=ORIENTED_EDGE ( 'NONE', *, *, #8254, .T. ) ;
#2822=ORIENTED_EDGE ( 'NONE', *, *, #8511, .F. ) ;
#2835=CARTESIAN_POINT ( 'NONE',  ( -26.64110105645932336, 8.000000000000000000, 125.0000000000000000 ) ) ;
#2839=CYLINDRICAL_SURFACE ( 'NONE', #1935, 11.99999999999983302 ) ;
#2850=ORIENTED_EDGE ( 'NONE', *, *, #8100, .T. ) ;
#2861=DIRECTION ( 'NONE',  ( -0.000000000000000000, -0.000000000000000000, -1.000000000000000000 ) ) ;
#2862=CYLINDRICAL_SURFACE ( 'NONE', #1208, 1.000000000000000888 ) ;
#2864=EDGE_LOOP ( 'NONE', ( #7292, #5058, #3473, #5473 ) ) ;
#2869=EDGE_LOOP ( 'NONE', ( #1443, #6359, #3501, #6514 ) ) ;
#2874=DIRECTION ( 'NONE',  ( -0.000000000000000000, -1.000000000000000000, -0.000000000000000000 ) ) ;
#2884=AXIS2_PLACEMENT_3D ( 'NONE', #118, #2157, #4842 ) ;
#2885=MANIFOLD_SOLID_BREP ( 'Fillet1', #527 ) ;
#2892=DIRECTION ( 'NONE',  ( 0.000000000000000000, 0.000000000000000000, -1.000000000000000000 ) ) ;
#2903=ORIENTED_EDGE ( 'NONE', *, *, #7411, .T. ) ;
#2905=DIRECTION ( 'NONE',  ( 0.000000000000000000, 0.000000000000000000, 1.000000000000000000 ) ) ;
#2910=ORIENTED_EDGE ( 'NONE', *, *, #2638, .F. ) ;
#2917=DIRECTION ( 'NONE',  ( 0.000000000000000000, 0.000000000000000000, 1.000000000000000000 ) ) ;
#2918=CARTESIAN_POINT ( 'NONE',  ( -30.00000000000002487, 0.000000000000000000, -44.00000000000000000 ) ) ;
#2926=DIRECTION ( 'NONE',  ( 1.000000000000000000, 0.000000000000000000, 0.000000000000000000 ) ) ;
#2932=CARTESIAN_POINT ( 'NONE',  ( -30.00000000000002842, 0.000000000000000000, -45.00000000000000000 ) ) ;
#2936=AXIS2_PLACEMENT_3D ( 'NONE', #830, #2917, #6911 ) ;
#2937=ORIENTED_EDGE ( 'NONE', *, *, #1822, .T. ) ;
#2945=CARTESIAN_POINT ( 'NONE',  ( -30.00000000000002487, 0.000000000000000000, -29.65000000000000213 ) ) ;
#2947=CARTESIAN_POINT ( 'NONE',  ( -34.35889894354067309, 8.000000000000000000, -24.00000000000000000 ) ) ;
#2950=EDGE_LOOP ( 'NONE', ( #6701, #824, #4740, #2164 ) ) ;
#2958=SPHERICAL_SURFACE ( 'NONE', #5145, 1.000000000000000000 ) ;
#2967=CARTESIAN_POINT ( 'NONE',  ( -33.35889894354067309, -7.999999999999996447, -23.99999999999999289 ) ) ;
#2983=ORIENTED_EDGE ( 'NONE', *, *, #893, .F. ) ;
#2994=ORIENTED_EDGE ( 'NONE', *, *, #7917, .F. ) ;
#2999=VECTOR ( 'NONE', #4748, 1000.000000000000000 ) ;
#3007=ORIENTED_EDGE ( 'NONE', *, *, #7941, .F. ) ;
#3009=EDGE_CURVE ( 'NONE', #5109, #1663, #1172, .T. ) ;
#3012=CIRCLE ( 'NONE', #2725, 12.00000000000000000 ) ;
#3020=EDGE_CURVE ( 'NONE', #2150, #3379, #4866, .T. ) ;
#3024=AXIS2_PLACEMENT_3D ( 'NONE', #1039, #4393, #8530 ) ;
#3028=ORIENTED_EDGE ( 'NONE', *, *, #1265, .T. ) ;
#3047=DIRECTION ( 'NONE',  ( 0.000000000000000000, 0.000000000000000000, -1.000000000000000000 ) ) ;
#3050=CYLINDRICAL_SURFACE ( 'NONE', #7494, 12.00000000000000000 ) ;
#3062=FACE_BOUND ( 'NONE', #7511, .T. ) ;
#3069=VERTEX_POINT ( 'NONE', #5180 ) ;
#3073=CIRCLE ( 'NONE', #5737, 1.000000000000000888 ) ;
#3077=CARTESIAN_POINT ( 'NONE',  ( -30.00000000000002487, 0.000000000000000000, -29.65000000000000213 ) ) ;
#3095=DIRECTION ( 'NONE',  ( -1.000000000000000000, -0.000000000000000000, 0.000000000000000000 ) ) ;
#3096=DIRECTION ( 'NONE',  ( -1.000000000000000000, 0.000000000000000000, 0.000000000000000000 ) ) ;
#3098=CARTESIAN_POINT ( 'NONE',  ( -40.00000000000002842, 1.224646799147353256E-15, -45.00000000000000000 ) ) ;
#3107=EDGE_LOOP ( 'NONE', ( #537, #4130, #8427, #2850 ) ) ;
#3115=CIRCLE ( 'NONE', #7328, 1.000000000000000888 ) ;
#3119=LINE ( 'NONE', #7119, #5124 ) ;
#3121=VERTEX_POINT ( 'NONE', #7248 ) ;
#3127=VERTEX_POINT ( 'NONE', #8535 ) ;
#3134=CARTESIAN_POINT ( 'NONE',  ( -30.00000000000002487, 0.000000000000000000, -28.65000000000000213 ) ) ;
#3146=ADVANCED_FACE ( 'NONE', ( #3249 ), #3297, .T. ) ;
#3160=CIRCLE ( 'NONE', #2884, 1.000000000000000888 ) ;
#3171=EDGE_LOOP ( 'NONE', ( #5856, #4703, #6154, #2983 ) ) ;
#3174=DIRECTION ( 'NONE',  ( -0.000000000000000000, -0.000000000000000000, -1.000000000000000000 ) ) ;
#3176=DIRECTION ( 'NONE',  ( -1.000000000000000000, 0.000000000000000000, 0.000000000000000000 ) ) ;
#3180=EDGE_LOOP ( 'NONE', ( #1965, #2795, #5234, #6820 ) ) ;
#3213=DIRECTION ( 'NONE',  ( -0.000000000000000000, -0.000000000000000000, -1.000000000000000000 ) ) ;
#3217=DIRECTION ( 'NONE',  ( 0.000000000000000000, 0.000000000000000000, 1.000000000000000000 ) ) ;
#3221=VERTEX_POINT ( 'NONE', #8495 ) ;
#3223=EDGE_CURVE ( 'NONE', #580, #3619, #6583, .T. ) ;
#3234=ORIENTED_EDGE ( 'NONE', *, *, #3542, .F. ) ;
#3239=CARTESIAN_POINT ( 'NONE',  ( -30.00000000000019185, 0.000000000000000000, -40.35000000000000142 ) ) ;
#3247=AXIS2_PLACEMENT_3D ( 'NONE', #276, #7591, #6841 ) ;
#3249=FACE_OUTER_BOUND ( 'NONE', #6089, .T. ) ;
#3259=EDGE_LOOP ( 'NONE', ( #3708, #7901 ) ) ;
#3271=PRODUCT_DEFINITION_FORMATION_WITH_SPECIFIED_SOURCE ( 'ANY', '', #2345, .NOT_KNOWN. ) ;
#3276=LINE ( 'NONE', #658, #7565 ) ;
#3277=EDGE_CURVE ( 'NONE', #1263, #2721, #6243, .T. ) ;
#3290=EDGE_CURVE ( 'NONE', #580, #3680, #8499, .T. ) ;
#3297=CYLINDRICAL_SURFACE ( 'NONE', #888, 1.000000000000000888 ) ;
#3311=EDGE_CURVE ( 'NONE', #3779, #3764, #8407, .T. ) ;
#3334=SURFACE_STYLE_FILL_AREA ( #3990 ) ;
#3342=ORIENTED_EDGE ( 'NONE', *, *, #6404, .T. ) ;
#3347=LINE ( 'NONE', #5268, #6368 ) ;
#3350=ORIENTED_EDGE ( 'NONE', *, *, #1007, .T. ) ;
#3361=CARTESIAN_POINT ( 'NONE',  ( -34.35889894354067309, 8.000000000000000000, 125.0000000000000000 ) ) ;
#3366=CARTESIAN_POINT ( 'NONE',  ( -30.00000000000002842, 0.000000000000000000, -26.00000000000000355 ) ) ;
#3373=CYLINDRICAL_SURFACE ( 'NONE', #4324, 11.99999999999979217 ) ;
#3376=DIRECTION ( 'NONE',  ( 0.000000000000000000, 0.000000000000000000, 1.000000000000000000 ) ) ;
#3377=DIRECTION ( 'NONE',  ( -0.000000000000000000, -0.000000000000000000, -1.000000000000000000 ) ) ;
#3379=VERTEX_POINT ( 'NONE', #6014 ) ;
#3386=ORIENTED_EDGE ( 'NONE', *, *, #6404, .F. ) ;
#3390=AXIS2_PLACEMENT_3D ( 'NONE', #2932, #5605, #5427 ) ;
#3408=CARTESIAN_POINT ( 'NONE',  ( -30.00000000000002487, 0.000000000000000000, -41.35000000000000142 ) ) ;
#3411=ADVANCED_FACE ( 'NONE', ( #5432 ), #4592, .F. ) ;
#3412=ORIENTED_EDGE ( 'NONE', *, *, #4868, .F. ) ;
#3431=VERTEX_POINT ( 'NONE', #6056 ) ;
#3433=STYLED_ITEM ( 'NONE', ( #7390 ), #2885 ) ;
#3434=( NAMED_UNIT ( * ) SI_UNIT ( $, .STERADIAN. ) SOLID_ANGLE_UNIT ( ) );
#3435=LINE ( 'NONE', #6110, #8616 ) ;
#3438=DIRECTION ( 'NONE',  ( 0.000000000000000000, 0.000000000000000000, 1.000000000000000000 ) ) ;
#3443=CARTESIAN_POINT ( 'NONE',  ( -40.00000000000002842, 1.224646799147353059E-15, -29.65000000000000213 ) ) ;
#3455=DIRECTION ( 'NONE',  ( 0.000000000000000000, 0.000000000000000000, -1.000000000000000000 ) ) ;
#3457=EDGE_LOOP ( 'NONE', ( #1896, #5800, #5419 ) ) ;
#3458=FACE_OUTER_BOUND ( 'NONE', #8186, .T. ) ;
#3466=VERTEX_POINT ( 'NONE', #6976 ) ;
#3468=ORIENTED_EDGE ( 'NONE', *, *, #5047, .F. ) ;
#3473=ORIENTED_EDGE ( 'NONE', *, *, #8303, .T. ) ;
#3481=ORIENTED_EDGE ( 'NONE', *, *, #3290, .T. ) ;
#3485=AXIS2_PLACEMENT_3D ( 'NONE', #1327, #5920, #4028 ) ;
#3486=ORIENTED_EDGE ( 'NONE', *, *, #5192, .F. ) ;
#3492=LINE ( 'NONE', #3649, #7759 ) ;
#3498=DIRECTION ( 'NONE',  ( 1.000000000000000000, 0.000000000000000000, 0.000000000000000000 ) ) ;
#3501=ORIENTED_EDGE ( 'NONE', *, *, #1007, .F. ) ;
#3511=EDGE_LOOP ( 'NONE', ( #7176, #8576, #8707 ) ) ;
#3517=EDGE_LOOP ( 'NONE', ( #1012, #5611 ) ) ;
#3542=EDGE_CURVE ( 'NONE', #6167, #2617, #6838, .T. ) ;
#3543=DIRECTION ( 'NONE',  ( -0.000000000000000000, -0.000000000000000000, -1.000000000000000000 ) ) ;
#3557=ADVANCED_FACE ( 'NONE', ( #4341 ), #932, .F. ) ;
#3564=CYLINDRICAL_SURFACE ( 'NONE', #8627, 12.00000000000004263 ) ;
#3565=LINE ( 'NONE', #5623, #6139 ) ;
#3569=CIRCLE ( 'NONE', #5780, 10.00000000000000178 ) ;
#3578=EDGE_LOOP ( 'NONE', ( #4886, #3735, #7957 ) ) ;
#3585=AXIS2_PLACEMENT_3D ( 'NONE', #1660, #7031, #4475 ) ;
#3590=ADVANCED_FACE ( 'NONE', ( #7594, #4914 ), #852, .F. ) ;
#3591=FACE_OUTER_BOUND ( 'NONE', #159, .T. ) ;
#3595=ORIENTED_EDGE ( 'NONE', *, *, #2699, .F. ) ;
#3597=ORIENTED_EDGE ( 'NONE', *, *, #441, .T. ) ;
#3604=DIRECTION ( 'NONE',  ( -0.000000000000000000, -0.000000000000000000, -1.000000000000000000 ) ) ;
#3605=AXIS2_PLACEMENT_3D ( 'NONE', #4334, #511, #7106 ) ;
#3614=FACE_OUTER_BOUND ( 'NONE', #6342, .T. ) ;
#3619=VERTEX_POINT ( 'NONE', #7687 ) ;
#3624=DIRECTION ( 'NONE',  ( -0.000000000000000000, -0.000000000000000000, -1.000000000000000000 ) ) ;
#3627=CIRCLE ( 'NONE', #1503, 11.99999999999983302 ) ;
#3647=CYLINDRICAL_SURFACE ( 'NONE', #3024, 1.000000000000000888 ) ;
#3649=CARTESIAN_POINT ( 'NONE',  ( -33.35889894354067309, -8.999999999999998224, 125.0000000000000000 ) ) ;
#3654=ORIENTED_EDGE ( 'NONE', *, *, #5197, .T. ) ;
#3664=EDGE_CURVE ( 'NONE', #7971, #3431, #2634, .T. ) ;
#3669=CARTESIAN_POINT ( 'NONE',  ( -30.00000000000002487, 0.000000000000000000, -44.00000000000000000 ) ) ;
#3672=FACE_OUTER_BOUND ( 'NONE', #7638, .T. ) ;
#3676=VECTOR ( 'NONE', #8345, 1000.000000000000000 ) ;
#3680=VERTEX_POINT ( 'NONE', #195 ) ;
#3688=DIRECTION ( 'NONE',  ( 1.000000000000000000, 0.000000000000000000, 0.000000000000000000 ) ) ;
#3692=DIRECTION ( 'NONE',  ( 1.000000000000000000, 0.000000000000000000, 0.000000000000000000 ) ) ;
#3700=DIRECTION ( 'NONE',  ( 1.000000000000000000, 0.000000000000000000, 0.000000000000000000 ) ) ;
#3702=DIRECTION ( 'NONE',  ( -0.000000000000000000, -0.000000000000000000, -1.000000000000000000 ) ) ;
#3708=ORIENTED_EDGE ( 'NONE', *, *, #4588, .F. ) ;
#3711=CARTESIAN_POINT ( 'NONE',  ( -25.64110105645932336, -7.999999999999996447, 125.0000000000000000 ) ) ;
#3723=ORIENTED_EDGE ( 'NONE', *, *, #8589, .F. ) ;
#3735=ORIENTED_EDGE ( 'NONE', *, *, #6983, .T. ) ;
#3741=CARTESIAN_POINT ( 'NONE',  ( -33.35889894354067309, 9.000000000000001776, 124.0000000000000000 ) ) ;
#3748=ORIENTED_EDGE ( 'NONE', *, *, #4949, .F. ) ;
#3758=CARTESIAN_POINT ( 'NONE',  ( -18.00000000000002132, 1.469576158976823947E-15, -29.65000000000000213 ) ) ;
#3759=CARTESIAN_POINT ( 'NONE',  ( -34.35889894354067309, -9.999999999999998224, -25.00000000000000000 ) ) ;
#3764=VERTEX_POINT ( 'NONE', #4202 ) ;
#3770=CIRCLE ( 'NONE', #2228, 10.00000000000000178 ) ;
#3779=VERTEX_POINT ( 'NONE', #6839 ) ;
#3787=CARTESIAN_POINT ( 'NONE',  ( -34.35889894354067309, 9.000000000000001776, -24.00000000000000000 ) ) ;
#3789=CARTESIAN_POINT ( 'NONE',  ( -30.00000000000002487, 0.000000000000000000, -28.65000000000000213 ) ) ;
#3804=EDGE_LOOP ( 'NONE', ( #1112, #5230, #5308, #2910 ) ) ;
#3809=CARTESIAN_POINT ( 'NONE',  ( -26.64110105645932336, -8.999999999999998224, 125.0000000000000000 ) ) ;
#3827=FACE_OUTER_BOUND ( 'NONE', #4439, .T. ) ;
#3839=AXIS2_PLACEMENT_3D ( 'NONE', #183, #2085, #5509 ) ;
#3840=VECTOR ( 'NONE', #5977, 1000.000000000000000 ) ;
#3843=CYLINDRICAL_SURFACE ( 'NONE', #6860, 1.000000000000000888 ) ;
#3852=AXIS2_PLACEMENT_3D ( 'NONE', #8618, #6668, #1164 ) ;
#3854=UNCERTAINTY_MEASURE_WITH_UNIT (LENGTH_MEASURE( 1.000000000000000082E-05 ), #8044, 'distance_accuracy_value', 'NONE');
#3858=DIRECTION ( 'NONE',  ( -0.000000000000000000, -0.000000000000000000, -1.000000000000000000 ) ) ;
#3873=CARTESIAN_POINT ( 'NONE',  ( -34.35889894354067309, -7.999999999999996447, 124.0000000000000000 ) ) ;
#3876=EDGE_LOOP ( 'NONE', ( #853, #123, #3386, #5247, #5128, #5637, #477, #4251 ) ) ;
#3879=EDGE_LOOP ( 'NONE', ( #1694, #5102, #7425, #4482 ) ) ;
#3882=DIRECTION ( 'NONE',  ( 1.000000000000000000, 0.000000000000000000, 0.000000000000000000 ) ) ;
#3891=ORIENTED_EDGE ( 'NONE', *, *, #2526, .T. ) ;
#3897=CARTESIAN_POINT ( 'NONE',  ( -34.35889894354067309, -7.999999999999996447, -24.00000000000000000 ) ) ;
#3908=ADVANCED_FACE ( 'NONE', ( #3591, #2141 ), #8266, .T. ) ;
#3909=AXIS2_PLACEMENT_3D ( 'NONE', #5281, #4066, #520 ) ;
#3916=PLANE ( 'NONE',  #315 ) ;
#3918=ADVANCED_FACE ( 'NONE', ( #4245 ), #229, .T. ) ;
#3922=EDGE_LOOP ( 'NONE', ( #5655, #6762, #2528, #7963 ) ) ;
#3923=CARTESIAN_POINT ( 'NONE',  ( -18.00000000000019185, 1.469576158976803042E-15, -40.35000000000000142 ) ) ;
#3954=SURFACE_SIDE_STYLE ('',( #4086 ) ) ;
#3959=ORIENTED_EDGE ( 'NONE', *, *, #8077, .F. ) ;
#3986=CARTESIAN_POINT ( 'NONE',  ( -20.00000000000002487, 0.000000000000000000, -28.65000000000000213 ) ) ;
#3990=FILL_AREA_STYLE ('',( #8575 ) ) ;
#3996=ORIENTED_EDGE ( 'NONE', *, *, #5318, .T. ) ;
#4000=CARTESIAN_POINT ( 'NONE',  ( -41.99999999999985789, 0.000000000000000000, -40.35000000000000142 ) ) ;
#4009=ORIENTED_EDGE ( 'NONE', *, *, #5197, .F. ) ;
#4020=DIRECTION ( 'NONE',  ( 0.000000000000000000, 0.000000000000000000, 1.000000000000000000 ) ) ;
#4028=DIRECTION ( 'NONE',  ( 1.000000000000000000, 0.000000000000000000, 0.000000000000000000 ) ) ;
#4033=CARTESIAN_POINT ( 'NONE',  ( -34.35889894354067309, 9.000000000000001776, 124.0000000000000000 ) ) ;
#4040=ORIENTED_EDGE ( 'NONE', *, *, #5163, .T. ) ;
#4049=EDGE_LOOP ( 'NONE', ( #7756, #1721, #8051, #4848 ) ) ;
#4058=AXIS2_PLACEMENT_3D ( 'NONE', #5867, #1861, #2399 ) ;
#4062=SHAPE_REPRESENTATION ( 'sliding jaw', ( #2554 ), #1987 ) ;
#4066=DIRECTION ( 'NONE',  ( 0.000000000000000000, 1.000000000000000000, 0.000000000000000000 ) ) ;
#4068=ORIENTED_EDGE ( 'NONE', *, *, #6250, .T. ) ;
#4086=SURFACE_STYLE_FILL_AREA ( #4706 ) ;
#4128=EDGE_CURVE ( 'NONE', #3779, #2752, #6046, .T. ) ;
#4129=ORIENTED_EDGE ( 'NONE', *, *, #8100, .F. ) ;
#4130=ORIENTED_EDGE ( 'NONE', *, *, #8544, .T. ) ;
#4144=AXIS2_PLACEMENT_3D ( 'NONE', #4695, #7380, #7507 ) ;
#4150=EDGE_CURVE ( 'NONE', #5443, #1195, #408, .T. ) ;
#4153=CYLINDRICAL_SURFACE ( 'NONE', #1587, 1.000000000000000888 ) ;
#4155=ORIENTED_EDGE ( 'NONE', *, *, #3542, .T. ) ;
#4175=FACE_OUTER_BOUND ( 'NONE', #4801, .T. ) ;
#4188=VECTOR ( 'NONE', #1243, 1000.000000000000000 ) ;
#4195=CYLINDRICAL_SURFACE ( 'NONE', #466, 10.00000000000000178 ) ;
#4199=EDGE_CURVE ( 'NONE', #5184, #1072, #5631, .T. ) ;
#4202=CARTESIAN_POINT ( 'NONE',  ( -26.64110105645932336, 9.000000000000001776, 124.0000000000000000 ) ) ;
#4206=EDGE_LOOP ( 'NONE', ( #6811, #2145, #3748, #812 ) ) ;
#4207=CARTESIAN_POINT ( 'NONE',  ( -30.00000000000002487, 0.000000000000000000, -25.00000000000000000 ) ) ;
#4212=ORIENTED_EDGE ( 'NONE', *, *, #5047, .T. ) ;
#4233=VECTOR ( 'NONE', #2892, 1000.000000000000000 ) ;
#4245=FACE_OUTER_BOUND ( 'NONE', #3107, .T. ) ;
#4251=ORIENTED_EDGE ( 'NONE', *, *, #3223, .T. ) ;
#4252=CARTESIAN_POINT ( 'NONE',  ( -29.99999999999998579, 0.000000000000000000, -26.00000000000000355 ) ) ;
#4268=CIRCLE ( 'NONE', #1608, 10.00000000000000178 ) ;
#4279=AXIS2_PLACEMENT_3D ( 'NONE', #4351, #952, #6325 ) ;
#4281=DIRECTION ( 'NONE',  ( 0.000000000000000000, 0.000000000000000000, -1.000000000000000000 ) ) ;
#4283=DIRECTION ( 'NONE',  ( 1.000000000000000000, 0.000000000000000000, 0.000000000000000000 ) ) ;
#4312=AXIS2_PLACEMENT_3D ( 'NONE', #1348, #3217, #8108 ) ;
#4324=AXIS2_PLACEMENT_3D ( 'NONE', #2710, #4691, #7907 ) ;
#4334=CARTESIAN_POINT ( 'NONE',  ( -30.00000000000002842, 0.000000000000000000, -45.00000000000000000 ) ) ;
#4341=FACE_OUTER_BOUND ( 'NONE', #8236, .T. ) ;
#4348=FACE_OUTER_BOUND ( 'NONE', #8270, .T. ) ;
#4351=CARTESIAN_POINT ( 'NONE',  ( -30.00000000000002842, 0.000000000000000000, -45.00000000000000000 ) ) ;
#4358=ORIENTED_EDGE ( 'NONE', *, *, #1723, .F. ) ;
#4367=EDGE_LOOP ( 'NONE', ( #6754, #7523, #1519, #4358 ) ) ;
#4368=APPLICATION_CONTEXT ( 'automotive_design' ) ;
#4372=LINE ( 'NONE', #4990, #6114 ) ;
#4373=CARTESIAN_POINT ( 'NONE',  ( -41.99999999999981526, 0.000000000000000000, -29.65000000000000213 ) ) ;
#4381=AXIS2_PLACEMENT_3D ( 'NONE', #7492, #4808, #1616 ) ;
#4390=FACE_OUTER_BOUND ( 'NONE', #3457, .T. ) ;
#4393=DIRECTION ( 'NONE',  ( 0.000000000000000000, -1.000000000000000000, 0.000000000000000000 ) ) ;
#4400=CIRCLE ( 'NONE', #7914, 2.000000000000001776 ) ;
#4408=VERTEX_POINT ( 'NONE', #714 ) ;
#4410=AXIS2_PLACEMENT_3D ( 'NONE', #6857, #4924, #5622 ) ;
#4412=ORIENTED_EDGE ( 'NONE', *, *, #5387, .T. ) ;
#4416=FACE_OUTER_BOUND ( 'NONE', #1427, .T. ) ;
#4418=DIRECTION ( 'NONE',  ( 0.000000000000000000, 0.000000000000000000, 1.000000000000000000 ) ) ;
#4421=CARTESIAN_POINT ( 'NONE',  ( -25.64110105645932336, -7.999999999999996447, -24.00000000000000000 ) ) ;
#4424=VECTOR ( 'NONE', #8001, 1000.000000000000000 ) ;
#4433=DIRECTION ( 'NONE',  ( 0.000000000000000000, 0.000000000000000000, -1.000000000000000000 ) ) ;
#4439=EDGE_LOOP ( 'NONE', ( #3959, #1388, #6582, #463 ) ) ;
#4461=CIRCLE ( 'NONE', #5869, 10.00000000000000178 ) ;
#4475=DIRECTION ( 'NONE',  ( 0.000000000000000000, 0.000000000000000000, -1.000000000000000000 ) ) ;
#4482=ORIENTED_EDGE ( 'NONE', *, *, #5318, .F. ) ;
#4486=CARTESIAN_POINT ( 'NONE',  ( -30.00000000000002487, 0.000000000000000000, -45.00000000000000000 ) ) ;
#4502=DIRECTION ( 'NONE',  ( 0.000000000000000000, 1.000000000000000000, -0.000000000000000000 ) ) ;
#4506=ORIENTED_EDGE ( 'NONE', *, *, #5477, .F. ) ;
#4511=VECTOR ( 'NONE', #3624, 1000.000000000000000 ) ;
#4516=LINE ( 'NONE', #4033, #4424 ) ;
#4525=VERTEX_POINT ( 'NONE', #7288 ) ;
#4540=DIRECTION ( 'NONE',  ( 0.000000000000000000, 0.000000000000000000, 1.000000000000000000 ) ) ;
#4546=EDGE_CURVE ( 'NONE', #2752, #3764, #2410, .T. ) ;
#4555=ADVANCED_FACE ( 'NONE', ( #6050 ), #8659, .T. ) ;
#4558=DIRECTION ( 'NONE',  ( -0.000000000000000000, -1.000000000000000000, 0.000000000000000000 ) ) ;
#4562=CARTESIAN_POINT ( 'NONE',  ( -30.00000000000002487, 0.000000000000000000, -26.00000000000000355 ) ) ;
#4571=VERTEX_POINT ( 'NONE', #3986 ) ;
#4574=DIRECTION ( 'NONE',  ( 0.000000000000000000, 0.000000000000000000, 1.000000000000000000 ) ) ;
#4581=EDGE_LOOP ( 'NONE', ( #4506, #3007 ) ) ;
#4585=DIRECTION ( 'NONE',  ( 0.000000000000000000, 0.000000000000000000, 1.000000000000000000 ) ) ;
#4586=TOROIDAL_SURFACE ( 'NONE', #8112, 2.000000000000000000, 1.000000000000000000 ) ;
#4588=EDGE_CURVE ( 'NONE', #1009, #2150, #7603, .T. ) ;
#4591=DIRECTION ( 'NONE',  ( 0.000000000000000000, 0.000000000000000000, 1.000000000000000000 ) ) ;
#4592=TOROIDAL_SURFACE ( 'NONE', #7693, 2.000000000000000000, 1.000000000000000000 ) ;
#4600=AXIS2_PLACEMENT_3D ( 'NONE', #1279, #1239, #5959 ) ;
#4601=LINE ( 'NONE', #7284, #4188 ) ;
#4608=CARTESIAN_POINT ( 'NONE',  ( -35.35889894354067309, 8.999999999999998224, -25.00000000000000000 ) ) ;
#4618=DIRECTION ( 'NONE',  ( 0.000000000000000000, 0.000000000000000000, 1.000000000000000000 ) ) ;
#4643=CARTESIAN_POINT ( 'NONE',  ( -33.35889894354067309, 8.000000000000000000, 124.0000000000000000 ) ) ;
#4654=ORIENTED_EDGE ( 'NONE', *, *, #4721, .F. ) ;
#4655=ORIENTED_EDGE ( 'NONE', *, *, #7880, .F. ) ;
#4657=DIRECTION ( 'NONE',  ( -0.000000000000000000, -0.000000000000000000, -1.000000000000000000 ) ) ;
#4662=AXIS2_PLACEMENT_3D ( 'NONE', #8473, #4540, #1775 ) ;
#4680=CYLINDRICAL_SURFACE ( 'NONE', #1508, 12.00000000000004263 ) ;
#4691=DIRECTION ( 'NONE',  ( -0.000000000000000000, -0.000000000000000000, -1.000000000000000000 ) ) ;
#4695=CARTESIAN_POINT ( 'NONE',  ( 0.000000000000000000, 0.000000000000000000, 125.0000000000000000 ) ) ;
#4703=ORIENTED_EDGE ( 'NONE', *, *, #7374, .T. ) ;
#4706=FILL_AREA_STYLE ('',( #2110 ) ) ;
#4707=CARTESIAN_POINT ( 'NONE',  ( -33.35889894354067309, 8.000000000000000000, -25.00000000000000000 ) ) ;
#4721=EDGE_CURVE ( 'NONE', #8337, #6952, #5653, .T. ) ;
#4728=ORIENTED_EDGE ( 'NONE', *, *, #1642, .F. ) ;
#4729=CARTESIAN_POINT ( 'NONE',  ( -20.00000000000002487, 0.000000000000000000, -26.00000000000000355 ) ) ;
#4740=ORIENTED_EDGE ( 'NONE', *, *, #7645, .T. ) ;
#4745=ORIENTED_EDGE ( 'NONE', *, *, #7374, .F. ) ;
#4748=DIRECTION ( 'NONE',  ( 0.000000000000000000, 0.000000000000000000, 1.000000000000000000 ) ) ;
#4752=AXIS2_PLACEMENT_3D ( 'NONE', #1930, #4657, #1345 ) ;
#4759=ORIENTED_EDGE ( 'NONE', *, *, #7035, .F. ) ;
#4763=AXIS2_PLACEMENT_3D ( 'NONE', #1779, #7854, #6523 ) ;
#4784=DIRECTION ( 'NONE',  ( 1.000000000000000000, 0.000000000000000000, 0.000000000000000000 ) ) ;
#4788=ORIENTED_EDGE ( 'NONE', *, *, #7138, .T. ) ;
#4792=DIRECTION ( 'NONE',  ( 0.000000000000000000, 0.000000000000000000, 1.000000000000000000 ) ) ;
#4795=DIRECTION ( 'NONE',  ( 0.000000000000000000, 0.000000000000000000, 1.000000000000000000 ) ) ;
#4801=EDGE_LOOP ( 'NONE', ( #3486, #725, #586, #2768 ) ) ;
#4808=DIRECTION ( 'NONE',  ( 1.000000000000000000, 0.000000000000000000, 0.000000000000000000 ) ) ;
#4820=AXIS2_PLACEMENT_3D ( 'NONE', #4707, #5311, #25 ) ;
#4842=DIRECTION ( 'NONE',  ( 1.000000000000000000, 0.000000000000000000, 0.000000000000000000 ) ) ;
#4844=ORIENTED_EDGE ( 'NONE', *, *, #4199, .F. ) ;
#4848=ORIENTED_EDGE ( 'NONE', *, *, #4949, .T. ) ;
#4860=CARTESIAN_POINT ( 'NONE',  ( -33.35889894354067309, 8.000000000000000000, 124.0000000000000000 ) ) ;
#4862=FACE_OUTER_BOUND ( 'NONE', #6947, .T. ) ;
#4866=LINE ( 'NONE', #5513, #5382 ) ;
#4868=EDGE_CURVE ( 'NONE', #1263, #3680, #7017, .T. ) ;
#4875=ORIENTED_EDGE ( 'NONE', *, *, #7155, .T. ) ;
#4882=FACE_OUTER_BOUND ( 'NONE', #2247, .T. ) ;
#4885=CARTESIAN_POINT ( 'NONE',  ( -30.00000000000002487, 0.000000000000000000, -26.00000000000000355 ) ) ;
#4886=ORIENTED_EDGE ( 'NONE', *, *, #1781, .T. ) ;
#4904=FACE_OUTER_BOUND ( 'NONE', #4206, .T. ) ;
#4908=CARTESIAN_POINT ( 'NONE',  ( -30.00000000000002842, 0.000000000000000000, -25.00000000000000000 ) ) ;
#4913=ORIENTED_EDGE ( 'NONE', *, *, #6300, .F. ) ;
#4914=FACE_OUTER_BOUND ( 'NONE', #1389, .T. ) ;
#4922=FACE_OUTER_BOUND ( 'NONE', #8378, .T. ) ;
#4924=DIRECTION ( 'NONE',  ( -0.000000000000000000, -0.000000000000000000, -1.000000000000000000 ) ) ;
#4926=EDGE_LOOP ( 'NONE', ( #6013, #4759, #673, #5538 ) ) ;
#4932=FACE_OUTER_BOUND ( 'NONE', #3511, .T. ) ;
#4936=ADVANCED_FACE ( 'NONE', ( #6356 ), #3843, .T. ) ;
#4943=DIRECTION ( 'NONE',  ( 1.000000000000000000, 0.000000000000000000, 0.000000000000000000 ) ) ;
#4945=CARTESIAN_POINT ( 'NONE',  ( -25.64110105645932336, 9.000000000000001776, 124.0000000000000000 ) ) ;
#4949=EDGE_CURVE ( 'NONE', #3069, #2202, #3073, .T. ) ;
#4956=VERTEX_POINT ( 'NONE', #1690 ) ;
#4966=LINE ( 'NONE', #7649, #8549 ) ;
#4970=CARTESIAN_POINT ( 'NONE',  ( -26.64110105645932336, 10.00000000000000178, -25.00000000000000000 ) ) ;
#4975=VECTOR ( 'NONE', #659, 1000.000000000000000 ) ;
#4982=DIRECTION ( 'NONE',  ( -1.000000000000000000, 0.000000000000000000, 0.000000000000000000 ) ) ;
#4990=CARTESIAN_POINT ( 'NONE',  ( -18.00000000000023093, 1.469576158976798506E-15, -29.65000000000000213 ) ) ;
#4991=AXIS2_PLACEMENT_3D ( 'NONE', #1321, #7010, #5689 ) ;
#5023=DIRECTION ( 'NONE',  ( -0.000000000000000000, -0.000000000000000000, -1.000000000000000000 ) ) ;
#5026=CIRCLE ( 'NONE', #7981, 1.000000000000000888 ) ;
#5032=DIRECTION ( 'NONE',  ( 0.000000000000000000, 0.000000000000000000, -1.000000000000000000 ) ) ;
#5039=DIRECTION ( 'NONE',  ( -1.000000000000000000, 0.000000000000000000, 0.000000000000000000 ) ) ;
#5042=VERTEX_POINT ( 'NONE', #8518 ) ;
#5047=EDGE_CURVE ( 'NONE', #2177, #598, #2484, .T. ) ;
#5051=DIRECTION ( 'NONE',  ( -1.000000000000000000, 0.000000000000000000, 0.000000000000000000 ) ) ;
#5058=ORIENTED_EDGE ( 'NONE', *, *, #6484, .T. ) ;
#5061=DIRECTION ( 'NONE',  ( -1.000000000000000000, -0.000000000000000000, -0.000000000000000000 ) ) ;
#5062=ADVANCED_FACE ( 'NONE', ( #1991 ), #4680, .T. ) ;
#5069=ORIENTED_EDGE ( 'NONE', *, *, #3009, .T. ) ;
#5073=DIRECTION ( 'NONE',  ( -0.000000000000000000, -0.000000000000000000, -1.000000000000000000 ) ) ;
#5074=PLANE ( 'NONE',  #8062 ) ;
#5078=FACE_OUTER_BOUND ( 'NONE', #3171, .T. ) ;
#5091=DIRECTION ( 'NONE',  ( 0.000000000000000000, -0.000000000000000000, 1.000000000000000000 ) ) ;
#5099=EDGE_CURVE ( 'NONE', #864, #2721, #7232, .T. ) ;
#5102=ORIENTED_EDGE ( 'NONE', *, *, #7524, .T. ) ;
#5106=DIRECTION ( 'NONE',  ( 1.000000000000000000, -0.000000000000000000, 0.000000000000000000 ) ) ;
#5109=VERTEX_POINT ( 'NONE', #7366 ) ;
#5112=VECTOR ( 'NONE', #4574, 1000.000000000000000 ) ;
#5117=DIRECTION ( 'NONE',  ( 0.000000000000000000, 0.000000000000000000, -1.000000000000000000 ) ) ;
#5124=VECTOR ( 'NONE', #5797, 1000.000000000000000 ) ;
#5128=ORIENTED_EDGE ( 'NONE', *, *, #3277, .F. ) ;
#5133=CARTESIAN_POINT ( 'NONE',  ( -33.35889894354067309, -7.999999999999996447, 124.0000000000000000 ) ) ;
#5145=AXIS2_PLACEMENT_3D ( 'NONE', #340, #6257, #3047 ) ;
#5147=DIRECTION ( 'NONE',  ( -1.000000000000000000, 0.000000000000000000, 0.000000000000000000 ) ) ;
#5162=AXIS2_PLACEMENT_3D ( 'NONE', #6159, #2197, #1522 ) ;
#5163=EDGE_CURVE ( 'NONE', #5681, #580, #6018, .T. ) ;
#5164=CARTESIAN_POINT ( 'NONE',  ( -25.64110105645932336, 9.000000000000001776, -24.00000000000000000 ) ) ;
#5165=CARTESIAN_POINT ( 'NONE',  ( -33.35889894354067309, -7.999999999999996447, 125.0000000000000000 ) ) ;
#5180=CARTESIAN_POINT ( 'NONE',  ( -33.35889894354067309, 9.000000000000001776, -24.00000000000000000 ) ) ;
#5184=VERTEX_POINT ( 'NONE', #563 ) ;
#5186=DIRECTION ( 'NONE',  ( -0.000000000000000000, -0.000000000000000000, -1.000000000000000000 ) ) ;
#5192=EDGE_CURVE ( 'NONE', #3431, #3121, #3276, .T. ) ;
#5197=EDGE_CURVE ( 'NONE', #1925, #6933, #3770, .T. ) ;
#5210=DIRECTION ( 'NONE',  ( 0.000000000000000000, 0.000000000000000000, -1.000000000000000000 ) ) ;
#5228=PLANE ( 'NONE',  #4312 ) ;
#5229=EDGE_CURVE ( 'NONE', #2721, #2177, #2791, .T. ) ;
#5230=ORIENTED_EDGE ( 'NONE', *, *, #5192, .T. ) ;
#5234=ORIENTED_EDGE ( 'NONE', *, *, #6999, .T. ) ;
#5235=CARTESIAN_POINT ( 'NONE',  ( -30.00000000000002487, 0.000000000000000000, -29.65000000000000213 ) ) ;
#5239=AXIS2_PLACEMENT_3D ( 'NONE', #7799, #7925, #6635 ) ;
#5245=DIRECTION ( 'NONE',  ( 0.000000000000000000, 0.000000000000000000, 1.000000000000000000 ) ) ;
#5247=ORIENTED_EDGE ( 'NONE', *, *, #5099, .T. ) ;
#5256=CARTESIAN_POINT ( 'NONE',  ( -25.64110105645932336, -8.999999999999998224, -24.00000000000000000 ) ) ;
#5263=EDGE_LOOP ( 'NONE', ( #2384, #2588, #8109, #3595 ) ) ;
#5268=CARTESIAN_POINT ( 'NONE',  ( -20.00000000000002487, 0.000000000000000000, -45.00000000000000000 ) ) ;
#5281=CARTESIAN_POINT ( 'NONE',  ( -24.64110105645932336, -7.999999999999996447, -24.00000000000000000 ) ) ;
#5287=CIRCLE ( 'NONE', #3485, 1.000000000000000888 ) ;
#5295=CARTESIAN_POINT ( 'NONE',  ( -26.64110105645932336, 8.000000000000000000, 124.0000000000000000 ) ) ;
#5308=ORIENTED_EDGE ( 'NONE', *, *, #1609, .F. ) ;
#5311=DIRECTION ( 'NONE',  ( 0.000000000000000000, 0.000000000000000000, 1.000000000000000000 ) ) ;
#5313=DIRECTION ( 'NONE',  ( 0.000000000000000000, -1.000000000000000000, 0.000000000000000000 ) ) ;
#5318=EDGE_CURVE ( 'NONE', #3379, #5895, #3627, .T. ) ;
#5332=DIRECTION ( 'NONE',  ( -0.000000000000000000, 1.000000000000000000, -0.000000000000000000 ) ) ;
#5343=DIRECTION ( 'NONE',  ( 0.000000000000000000, 0.000000000000000000, -1.000000000000000000 ) ) ;
#5347=AXIS2_PLACEMENT_3D ( 'NONE', #2396, #973, #2926 ) ;
#5355=ADVANCED_FACE ( 'NONE', ( #4348 ), #7825, .T. ) ;
#5366=LINE ( 'NONE', #3361, #1554 ) ;
#5372=LINE ( 'NONE', #6743, #4975 ) ;
#5382=VECTOR ( 'NONE', #3543, 1000.000000000000000 ) ;
#5387=EDGE_CURVE ( 'NONE', #5042, #112, #2364, .T. ) ;
#5391=VECTOR ( 'NONE', #1877, 1000.000000000000000 ) ;
#5396=CARTESIAN_POINT ( 'NONE',  ( -20.00000000000002487, 0.000000000000000000, -45.00000000000000000 ) ) ;
#5400=ORIENTED_EDGE ( 'NONE', *, *, #3664, .F. ) ;
#5405=VERTEX_POINT ( 'NONE', #989 ) ;
#5419=ORIENTED_EDGE ( 'NONE', *, *, #771, .F. ) ;
#5427=DIRECTION ( 'NONE',  ( 1.000000000000000000, 0.000000000000000000, 0.000000000000000000 ) ) ;
#5432=FACE_OUTER_BOUND ( 'NONE', #4049, .T. ) ;
#5439=DIRECTION ( 'NONE',  ( 1.000000000000000000, -0.000000000000000000, -0.000000000000000000 ) ) ;
#5443=VERTEX_POINT ( 'NONE', #8487 ) ;
#5444=VECTOR ( 'NONE', #7275, 1000.000000000000000 ) ;
#5451=LINE ( 'NONE', #964, #6225 ) ;
#5454=ADVANCED_FACE ( 'NONE', ( #4390 ), #6366, .T. ) ;
#5461=CARTESIAN_POINT ( 'NONE',  ( -18.00000000000023093, 1.469576158976798506E-15, -44.00000000000000000 ) ) ;
#5463=EDGE_LOOP ( 'NONE', ( #4728, #2406, #7595, #4913 ) ) ;
#5464=FACE_OUTER_BOUND ( 'NONE', #6498, .T. ) ;
#5473=ORIENTED_EDGE ( 'NONE', *, *, #2565, .F. ) ;
#5475=VERTEX_POINT ( 'NONE', #1117 ) ;
#5477=EDGE_CURVE ( 'NONE', #5715, #8141, #96, .T. ) ;
#5487=AXIS2_PLACEMENT_3D ( 'NONE', #5295, #3376, #8091 ) ;
#5489=DIRECTION ( 'NONE',  ( -1.000000000000000000, 0.000000000000000000, 0.000000000000000000 ) ) ;
#5502=EDGE_CURVE ( 'NONE', #6167, #8337, #1647, .T. ) ;
#5509=DIRECTION ( 'NONE',  ( 0.000000000000000000, 0.000000000000000000, 1.000000000000000000 ) ) ;
#5513=CARTESIAN_POINT ( 'NONE',  ( -18.00000000000019185, 1.469576158976803042E-15, -29.65000000000000213 ) ) ;
#5534=DIRECTION ( 'NONE',  ( -1.000000000000000000, 0.000000000000000000, 0.000000000000000000 ) ) ;
#5536=DIRECTION ( 'NONE',  ( -1.000000000000000000, 0.000000000000000000, 0.000000000000000000 ) ) ;
#5538=ORIENTED_EDGE ( 'NONE', *, *, #5756, .F. ) ;
#5554=CYLINDRICAL_SURFACE ( 'NONE', #4991, 1.000000000000000888 ) ;
#5562=DIRECTION ( 'NONE',  ( 1.000000000000000000, 0.000000000000000000, 0.000000000000000000 ) ) ;
#5574=FACE_BOUND ( 'NONE', #7095, .T. ) ;
#5596=CIRCLE ( 'NONE', #2936, 1.000000000000000888 ) ;
#5605=DIRECTION ( 'NONE',  ( 0.000000000000000000, 0.000000000000000000, 1.000000000000000000 ) ) ;
#5611=ORIENTED_EDGE ( 'NONE', *, *, #6484, .F. ) ;
#5613=ADVANCED_FACE ( 'NONE', ( #8569 ), #3373, .T. ) ;
#5622=DIRECTION ( 'NONE',  ( 1.000000000000000000, 0.000000000000000000, 0.000000000000000000 ) ) ;
#5623=CARTESIAN_POINT ( 'NONE',  ( -20.00000000000002487, 0.000000000000000000, -45.00000000000000000 ) ) ;
#5631=CIRCLE ( 'NONE', #6470, 12.00000000000000000 ) ;
#5635=CARTESIAN_POINT ( 'NONE',  ( -26.64110105645932336, 8.000000000000000000, -25.00000000000000000 ) ) ;
#5637=ORIENTED_EDGE ( 'NONE', *, *, #4868, .T. ) ;
#5649=DIRECTION ( 'NONE',  ( 0.000000000000000000, 0.000000000000000000, 1.000000000000000000 ) ) ;
#5651=CARTESIAN_POINT ( 'NONE',  ( -26.64110105645932336, 8.000000000000000000, 124.0000000000000000 ) ) ;
#5653=LINE ( 'NONE', #7506, #4233 ) ;
#5655=ORIENTED_EDGE ( 'NONE', *, *, #3277, .T. ) ;
#5657=ORIENTED_EDGE ( 'NONE', *, *, #7332, .F. ) ;
#5665=CIRCLE ( 'NONE', #5239, 10.00000000000000178 ) ;
#5681=VERTEX_POINT ( 'NONE', #3897 ) ;
#5689=DIRECTION ( 'NONE',  ( 0.000000000000000000, 0.000000000000000000, 1.000000000000000000 ) ) ;
#5691=EDGE_CURVE ( 'NONE', #999, #1072, #4601, .T. ) ;
#5707=CARTESIAN_POINT ( 'NONE',  ( -30.00000000000002842, 0.000000000000000000, -26.00000000000000355 ) ) ;
#5715=VERTEX_POINT ( 'NONE', #4729 ) ;
#5718=ORIENTED_EDGE ( 'NONE', *, *, #441, .F. ) ;
#5724=CYLINDRICAL_SURFACE ( 'NONE', #6784, 11.99999999999983302 ) ;
#5727=VECTOR ( 'NONE', #6450, 1000.000000000000000 ) ;
#5730=ORIENTED_EDGE ( 'NONE', *, *, #7035, .T. ) ;
#5737=AXIS2_PLACEMENT_3D ( 'NONE', #8479, #1782, #7682 ) ;
#5739=PLANE ( 'NONE',  #4763 ) ;
#5756=EDGE_CURVE ( 'NONE', #1195, #3779, #2041, .T. ) ;
#5757=DIRECTION ( 'NONE',  ( 0.000000000000000000, 0.000000000000000000, -1.000000000000000000 ) ) ;
#5767=CARTESIAN_POINT ( 'NONE',  ( -30.00000000000002487, 0.000000000000000000, -29.65000000000000213 ) ) ;
#5779=DIRECTION ( 'NONE',  ( 0.000000000000000000, 0.000000000000000000, 1.000000000000000000 ) ) ;
#5780=AXIS2_PLACEMENT_3D ( 'NONE', #1545, #2311, #4283 ) ;
#5791=( GEOMETRIC_REPRESENTATION_CONTEXT ( 3 ) GLOBAL_UNCERTAINTY_ASSIGNED_CONTEXT ( ( #7028 ) ) GLOBAL_UNIT_ASSIGNED_CONTEXT ( ( #6053, #2005, #6714 ) ) REPRESENTATION_CONTEXT ( 'NONE', 'WORKASPACE' ) );
#5792=ADVANCED_FACE ( 'NONE', ( #3458 ), #6090, .F. ) ;
#5793=UNCERTAINTY_MEASURE_WITH_UNIT (LENGTH_MEASURE( 1.000000000000000082E-05 ), #590, 'distance_accuracy_value', 'NONE');
#5794=DIRECTION ( 'NONE',  ( 1.000000000000000000, 0.000000000000000000, 0.000000000000000000 ) ) ;
#5797=DIRECTION ( 'NONE',  ( 0.000000000000000000, -1.000000000000000000, -0.000000000000000000 ) ) ;
#5800=ORIENTED_EDGE ( 'NONE', *, *, #8511, .T. ) ;
#5820=PRODUCT_DEFINITION_CONTEXT ( 'detailed design', #6951, 'design' ) ;
#5822=AXIS2_PLACEMENT_3D ( 'NONE', #59, #7336, #2053 ) ;
#5852=DIRECTION ( 'NONE',  ( -1.000000000000000000, 0.000000000000000000, 0.000000000000000000 ) ) ;
#5856=ORIENTED_EDGE ( 'NONE', *, *, #1157, .T. ) ;
#5867=CARTESIAN_POINT ( 'NONE',  ( -24.64110105645932336, 8.000000000000000000, -24.00000000000000000 ) ) ;
#5869=AXIS2_PLACEMENT_3D ( 'NONE', #162, #2905, #5534 ) ;
#5879=ADVANCED_FACE ( 'NONE', ( #5464 ), #2839, .T. ) ;
#5882=DIRECTION ( 'NONE',  ( 0.000000000000000000, 0.000000000000000000, 1.000000000000000000 ) ) ;
#5887=CARTESIAN_POINT ( 'NONE',  ( -30.00000000000002487, 0.000000000000000000, -40.35000000000000142 ) ) ;
#5889=PRODUCT_DEFINITION ( 'UNKNOWN', '', #3271, #5820 ) ;
#5895=VERTEX_POINT ( 'NONE', #6351 ) ;
#5913=CARTESIAN_POINT ( 'NONE',  ( -30.00000000000002487, 0.000000000000000000, -29.65000000000000213 ) ) ;
#5920=DIRECTION ( 'NONE',  ( -0.000000000000000000, 0.000000000000000000, 1.000000000000000000 ) ) ;
#5935=DIRECTION ( 'NONE',  ( -0.000000000000000000, -0.000000000000000000, 1.000000000000000000 ) ) ;
#5942=CIRCLE ( 'NONE', #4820, 2.000000000000001776 ) ;
#5949=AXIS2_PLACEMENT_3D ( 'NONE', #2245, #6945, #1394 ) ;
#5955=DIRECTION ( 'NONE',  ( -1.000000000000000000, 0.000000000000000000, 0.000000000000000000 ) ) ;
#5959=DIRECTION ( 'NONE',  ( 0.000000000000000000, 0.000000000000000000, 1.000000000000000000 ) ) ;
#5977=DIRECTION ( 'NONE',  ( -0.000000000000000000, -0.000000000000000000, 1.000000000000000000 ) ) ;
#5991=CARTESIAN_POINT ( 'NONE',  ( -33.35889894354067309, -7.999999999999996447, 124.0000000000000000 ) ) ;
#6012=PRESENTATION_STYLE_ASSIGNMENT (( #6670 ) ) ;
#6013=ORIENTED_EDGE ( 'NONE', *, *, #6983, .F. ) ;
#6014=CARTESIAN_POINT ( 'NONE',  ( -18.00000000000019185, 1.469576158976803042E-15, -41.35000000000000142 ) ) ;
#6018=CIRCLE ( 'NONE', #2649, 1.000000000000000888 ) ;
#6046=CIRCLE ( 'NONE', #8454, 1.000000000000000888 ) ;
#6050=FACE_OUTER_BOUND ( 'NONE', #360, .T. ) ;
#6051=DIRECTION ( 'NONE',  ( -1.000000000000000000, 0.000000000000000000, 0.000000000000000000 ) ) ;
#6053=( LENGTH_UNIT ( ) NAMED_UNIT ( * ) SI_UNIT ( .MILLI., .METRE. ) );
#6056=CARTESIAN_POINT ( 'NONE',  ( -17.99999999999998579, 1.469576158976828483E-15, -25.00000000000000000 ) ) ;
#6089=EDGE_LOOP ( 'NONE', ( #8297, #5657, #8715, #194 ) ) ;
#6090=CYLINDRICAL_SURFACE ( 'NONE', #4600, 1.000000000000000888 ) ;
#6105=ORIENTED_EDGE ( 'NONE', *, *, #3009, .F. ) ;
#6109=CARTESIAN_POINT ( 'NONE',  ( -24.64110105645932336, -7.999999999999996447, -25.00000000000000000 ) ) ;
#6110=CARTESIAN_POINT ( 'NONE',  ( -25.64110105645932336, -7.999999999999996447, 125.0000000000000000 ) ) ;
#6114=VECTOR ( 'NONE', #7102, 1000.000000000000000 ) ;
#6115=ADVANCED_FACE ( 'NONE', ( #6395 ), #7143, .T. ) ;
#6133=CARTESIAN_POINT ( 'NONE',  ( -30.00000000000002842, 0.000000000000000000, -45.00000000000000000 ) ) ;
#6134=PRODUCT_CONTEXT ( 'NONE', #4368, 'mechanical' ) ;
#6139=VECTOR ( 'NONE', #2246, 1000.000000000000000 ) ;
#6154=ORIENTED_EDGE ( 'NONE', *, *, #7941, .T. ) ;
#6158=EDGE_CURVE ( 'NONE', #4956, #4525, #6519, .T. ) ;
#6159=CARTESIAN_POINT ( 'NONE',  ( -33.35889894354067309, -7.999999999999996447, 125.0000000000000000 ) ) ;
#6162=DIRECTION ( 'NONE',  ( 0.000000000000000000, 0.000000000000000000, -1.000000000000000000 ) ) ;
#6164=VECTOR ( 'NONE', #4502, 1000.000000000000000 ) ;
#6167=VERTEX_POINT ( 'NONE', #471 ) ;
#6172=CYLINDRICAL_SURFACE ( 'NONE', #2436, 10.00000000000000178 ) ;
#6200=DIRECTION ( 'NONE',  ( -0.000000000000000000, -0.000000000000000000, 1.000000000000000000 ) ) ;
#6214=COLOUR_RGB ( '', 0.31764706, 0.68627451, 0.89019608) ;
#6220=FACE_OUTER_BOUND ( 'NONE', #5263, .T. ) ;
#6225=VECTOR ( 'NONE', #2874, 1000.000000000000000 ) ;
#6240=ADVANCED_FACE ( 'NONE', ( #8557 ), #5074, .T. ) ;
#6243=CIRCLE ( 'NONE', #7363, 2.000000000000001776 ) ;
#6250=EDGE_CURVE ( 'NONE', #6933, #5109, #431, .T. ) ;
#6254=ORIENTED_EDGE ( 'NONE', *, *, #1189, .F. ) ;
#6257=DIRECTION ( 'NONE',  ( -0.000000000000000000, 1.000000000000000000, 0.000000000000000000 ) ) ;
#6258=CIRCLE ( 'NONE', #6949, 12.00000000000004263 ) ;
#6295=AXIS2_PLACEMENT_3D ( 'NONE', #1612, #7602, #8322 ) ;
#6298=AXIS2_PLACEMENT_3D ( 'NONE', #8695, #4558, #5882 ) ;
#6300=EDGE_CURVE ( 'NONE', #6952, #5681, #5451, .T. ) ;
#6305=DIRECTION ( 'NONE',  ( 1.000000000000000000, 0.000000000000000000, 0.000000000000000000 ) ) ;
#6307=CARTESIAN_POINT ( 'NONE',  ( -34.35889894354067309, 8.000000000000000000, 124.0000000000000000 ) ) ;
#6311=FACE_OUTER_BOUND ( 'NONE', #3922, .T. ) ;
#6317=EDGE_LOOP ( 'NONE', ( #7439, #1757, #2822, #6254 ) ) ;
#6318=DIRECTION ( 'NONE',  ( 1.000000000000000000, 0.000000000000000000, -0.000000000000000000 ) ) ;
#6325=DIRECTION ( 'NONE',  ( 1.000000000000000000, 0.000000000000000000, 0.000000000000000000 ) ) ;
#6341=EDGE_CURVE ( 'NONE', #4956, #7944, #6782, .T. ) ;
#6342=EDGE_LOOP ( 'NONE', ( #1183, #4788, #8708, #4412 ) ) ;
#6343=PRODUCT_DEFINITION_SHAPE ( 'NONE', 'NONE',  #5889 ) ;
#6349=ADVANCED_FACE ( 'NONE', ( #2168 ), #6172, .T. ) ;
#6351=CARTESIAN_POINT ( 'NONE',  ( -41.99999999999985789, 0.000000000000000000, -41.35000000000000142 ) ) ;
#6356=FACE_OUTER_BOUND ( 'NONE', #4367, .T. ) ;
#6358=CIRCLE ( 'NONE', #2567, 1.000000000000000888 ) ;
#6359=ORIENTED_EDGE ( 'NONE', *, *, #8077, .T. ) ;
#6360=ORIENTED_EDGE ( 'NONE', *, *, #2565, .T. ) ;
#6365=CARTESIAN_POINT ( 'NONE',  ( -33.35889894354067309, -8.999999999999998224, 124.0000000000000000 ) ) ;
#6366=SPHERICAL_SURFACE ( 'NONE', #2505, 1.000000000000000000 ) ;
#6368=VECTOR ( 'NONE', #4618, 1000.000000000000000 ) ;
#6373=ORIENTED_EDGE ( 'NONE', *, *, #5756, .T. ) ;
#6377=ORIENTED_EDGE ( 'NONE', *, *, #7702, .T. ) ;
#6395=FACE_OUTER_BOUND ( 'NONE', #6317, .T. ) ;
#6399=DIRECTION ( 'NONE',  ( 1.000000000000000000, 0.000000000000000000, 0.000000000000000000 ) ) ;
#6404=EDGE_CURVE ( 'NONE', #864, #8551, #4400, .T. ) ;
#6410=DIRECTION ( 'NONE',  ( -0.000000000000000000, 1.000000000000000000, 0.000000000000000000 ) ) ;
#6424=DIRECTION ( 'NONE',  ( -1.000000000000000000, 0.000000000000000000, 0.000000000000000000 ) ) ;
#6427=DIRECTION ( 'NONE',  ( -1.000000000000000000, 0.000000000000000000, 0.000000000000000000 ) ) ;
#6430=CIRCLE ( 'NONE', #1926, 12.00000000000004263 ) ;
#6437=CARTESIAN_POINT ( 'NONE',  ( -42.00000000000002132, 0.000000000000000000, -29.65000000000000213 ) ) ;
#6438=EDGE_CURVE ( 'NONE', #5475, #999, #7777, .T. ) ;
#6441=CYLINDRICAL_SURFACE ( 'NONE', #3605, 10.00000000000000178 ) ;
#6443=DIRECTION ( 'NONE',  ( -1.000000000000000000, 0.000000000000000000, 0.000000000000000000 ) ) ;
#6450=DIRECTION ( 'NONE',  ( -0.000000000000000000, -0.000000000000000000, 1.000000000000000000 ) ) ;
#6464=PLANE ( 'NONE',  #8491 ) ;
#6470=AXIS2_PLACEMENT_3D ( 'NONE', #3077, #3858, #5051 ) ;
#6478=AXIS2_PLACEMENT_3D ( 'NONE', #82, #2789, #8025 ) ;
#6484=EDGE_CURVE ( 'NONE', #999, #5475, #2715, .T. ) ;
#6498=EDGE_LOOP ( 'NONE', ( #1537, #450, #7613, #2994 ) ) ;
#6501=ADVANCED_FACE ( 'NONE', ( #1094 ), #3050, .T. ) ;
#6502=ORIENTED_EDGE ( 'NONE', *, *, #6999, .F. ) ;
#6506=LINE ( 'NONE', #1177, #1735 ) ;
#6507=CYLINDRICAL_SURFACE ( 'NONE', #7490, 11.99999999999979217 ) ;
#6511=AXIS2_PLACEMENT_3D ( 'NONE', #3366, #2750, #3498 ) ;
#6514=ORIENTED_EDGE ( 'NONE', *, *, #6158, .F. ) ;
#6516=AXIS2_PLACEMENT_3D ( 'NONE', #2196, #6985, #3688 ) ;
#6519=LINE ( 'NONE', #4373, #2154 ) ;
#6523=DIRECTION ( 'NONE',  ( -1.000000000000000000, 0.000000000000000000, 0.000000000000000000 ) ) ;
#6538=CARTESIAN_POINT ( 'NONE',  ( -40.00000000000002842, 1.224646799147353256E-15, -45.00000000000000000 ) ) ;
#6540=ORIENTED_EDGE ( 'NONE', *, *, #5387, .F. ) ;
#6582=ORIENTED_EDGE ( 'NONE', *, *, #6158, .T. ) ;
#6583=LINE ( 'NONE', #4608, #1744 ) ;
#6598=ADVANCED_FACE ( 'NONE', ( #419 ), #5724, .T. ) ;
#6612=ORIENTED_EDGE ( 'NONE', *, *, #5502, .F. ) ;
#6622=SURFACE_SIDE_STYLE ('',( #3334 ) ) ;
#6631=SURFACE_STYLE_USAGE ( .BOTH. , #3954 ) ;
#6635=DIRECTION ( 'NONE',  ( -1.000000000000000000, 0.000000000000000000, 0.000000000000000000 ) ) ;
#6640=AXIS2_PLACEMENT_3D ( 'NONE', #8515, #644, #391 ) ;
#6648=( GEOMETRIC_REPRESENTATION_CONTEXT ( 3 ) GLOBAL_UNCERTAINTY_ASSIGNED_CONTEXT ( ( #5793 ) ) GLOBAL_UNIT_ASSIGNED_CONTEXT ( ( #590, #1300, #3434 ) ) REPRESENTATION_CONTEXT ( 'NONE', 'WORKASPACE' ) );
#6668=DIRECTION ( 'NONE',  ( 0.000000000000000000, 0.000000000000000000, -1.000000000000000000 ) ) ;
#6670=SURFACE_STYLE_USAGE ( .BOTH. , #6622 ) ;
#6671=ORIENTED_EDGE ( 'NONE', *, *, #8524, .F. ) ;
#6684=ORIENTED_EDGE ( 'NONE', *, *, #1265, .F. ) ;
#6700=FACE_OUTER_BOUND ( 'NONE', #595, .T. ) ;
#6701=ORIENTED_EDGE ( 'NONE', *, *, #1189, .T. ) ;
#6705=CIRCLE ( 'NONE', #4752, 11.99999999999979217 ) ;
#6714=( NAMED_UNIT ( * ) SI_UNIT ( $, .STERADIAN. ) SOLID_ANGLE_UNIT ( ) );
#6728=FACE_OUTER_BOUND ( 'NONE', #1486, .T. ) ;
#6743=CARTESIAN_POINT ( 'NONE',  ( -41.99999999999985789, 0.000000000000000000, -29.65000000000000213 ) ) ;
#6744=EDGE_LOOP ( 'NONE', ( #7842, #1215 ) ) ;
#6749=DIRECTION ( 'NONE',  ( -1.000000000000000000, 0.000000000000000000, 0.000000000000000000 ) ) ;
#6754=ORIENTED_EDGE ( 'NONE', *, *, #7148, .T. ) ;
#6762=ORIENTED_EDGE ( 'NONE', *, *, #5229, .T. ) ;
#6766=CARTESIAN_POINT ( 'NONE',  ( -25.64110105645932336, 10.00000000000000178, -25.00000000000000000 ) ) ;
#6769=EDGE_CURVE ( 'NONE', #3127, #4571, #5665, .T. ) ;
#6782=CIRCLE ( 'NONE', #8213, 11.99999999999979217 ) ;
#6784=AXIS2_PLACEMENT_3D ( 'NONE', #8545, #3702, #6427 ) ;
#6787=DIRECTION ( 'NONE',  ( 0.000000000000000000, 0.000000000000000000, 1.000000000000000000 ) ) ;
#6810=AXIS2_PLACEMENT_3D ( 'NONE', #822, #4795, #776 ) ;
#6811=ORIENTED_EDGE ( 'NONE', *, *, #8589, .T. ) ;
#6820=ORIENTED_EDGE ( 'NONE', *, *, #1464, .F. ) ;
#6831=CARTESIAN_POINT ( 'NONE',  ( -42.00000000000006395, 0.000000000000000000, -25.00000000000000000 ) ) ;
#6833=EDGE_LOOP ( 'NONE', ( #4129, #6105 ) ) ;
#6838=CIRCLE ( 'NONE', #7263, 1.000000000000000888 ) ;
#6839=CARTESIAN_POINT ( 'NONE',  ( -26.64110105645932336, 8.000000000000000000, 125.0000000000000000 ) ) ;
#6841=DIRECTION ( 'NONE',  ( -1.000000000000000000, 0.000000000000000000, 0.000000000000000000 ) ) ;
#6843=VECTOR ( 'NONE', #5210, 1000.000000000000000 ) ;
#6851=AXIS2_PLACEMENT_3D ( 'NONE', #1830, #6410, #5091 ) ;
#6857=CARTESIAN_POINT ( 'NONE',  ( -30.00000000000002842, 0.000000000000000000, -29.65000000000000213 ) ) ;
#6860=AXIS2_PLACEMENT_3D ( 'NONE', #319, #396, #5039 ) ;
#6891=ADVANCED_FACE ( 'NONE', ( #1219 ), #3916, .T. ) ;
#6907=EDGE_LOOP ( 'NONE', ( #8228, #2806, #1472, #4875 ) ) ;
#6911=DIRECTION ( 'NONE',  ( 1.000000000000000000, 0.000000000000000000, 0.000000000000000000 ) ) ;
#6917=CARTESIAN_POINT ( 'NONE',  ( -26.64110105645932336, -9.999999999999998224, -25.00000000000000000 ) ) ;
#6920=DIRECTION ( 'NONE',  ( 1.000000000000000000, -0.000000000000000000, 0.000000000000000000 ) ) ;
#6921=EDGE_CURVE ( 'NONE', #1925, #1663, #3347, .T. ) ;
#6923=DIRECTION ( 'NONE',  ( -0.000000000000000000, -0.000000000000000000, -1.000000000000000000 ) ) ;
#6925=AXIS2_PLACEMENT_3D ( 'NONE', #3134, #303, #3176 ) ;
#6933=VERTEX_POINT ( 'NONE', #8713 ) ;
#6945=DIRECTION ( 'NONE',  ( 0.000000000000000000, -1.000000000000000000, 0.000000000000000000 ) ) ;
#6947=EDGE_LOOP ( 'NONE', ( #1934, #2278, #3234, #6671 ) ) ;
#6949=AXIS2_PLACEMENT_3D ( 'NONE', #4562, #3377, #6051 ) ;
#6951=APPLICATION_CONTEXT ( 'automotive_design' ) ;
#6952=VERTEX_POINT ( 'NONE', #2947 ) ;
#6961=ADVANCED_FACE ( 'NONE', ( #4175 ), #3564, .T. ) ;
#6964=CARTESIAN_POINT ( 'NONE',  ( -26.64110105645932336, -7.999999999999996447, 124.0000000000000000 ) ) ;
#6976=CARTESIAN_POINT ( 'NONE',  ( -42.00000000000006395, 0.000000000000000000, -26.00000000000000355 ) ) ;
#6983=EDGE_CURVE ( 'NONE', #3221, #1195, #1021, .T. ) ;
#6985=DIRECTION ( 'NONE',  ( -0.000000000000000000, -0.000000000000000000, -1.000000000000000000 ) ) ;
#6988=FACE_OUTER_BOUND ( 'NONE', #5463, .T. ) ;
#6999=EDGE_CURVE ( 'NONE', #112, #5042, #2162, .T. ) ;
#7008=CARTESIAN_POINT ( 'NONE',  ( -30.00000000000002842, -9.999999999999998224, -24.00000000000000000 ) ) ;
#7010=DIRECTION ( 'NONE',  ( -1.000000000000000000, 0.000000000000000000, 0.000000000000000000 ) ) ;
#7014=DIRECTION ( 'NONE',  ( 0.000000000000000000, 1.000000000000000000, 0.000000000000000000 ) ) ;
#7017=LINE ( 'NONE', #3759, #1654 ) ;
#7028=UNCERTAINTY_MEASURE_WITH_UNIT (LENGTH_MEASURE( 1.000000000000000082E-05 ), #6053, 'distance_accuracy_value', 'NONE');
#7031=DIRECTION ( 'NONE',  ( -0.000000000000000000, 1.000000000000000000, 0.000000000000000000 ) ) ;
#7034=EDGE_LOOP ( 'NONE', ( #6540, #6502 ) ) ;
#7035=EDGE_CURVE ( 'NONE', #2752, #3221, #1567, .T. ) ;
#7045=EDGE_CURVE ( 'NONE', #2202, #8551, #909, .T. ) ;
#7095=EDGE_LOOP ( 'NONE', ( #4009, #2159 ) ) ;
#7102=DIRECTION ( 'NONE',  ( -0.000000000000000000, -0.000000000000000000, -1.000000000000000000 ) ) ;
#7106=DIRECTION ( 'NONE',  ( 1.000000000000000000, 0.000000000000000000, 0.000000000000000000 ) ) ;
#7119=CARTESIAN_POINT ( 'NONE',  ( -33.35889894354067309, -8.999999999999998224, 125.0000000000000000 ) ) ;
#7129=LINE ( 'NONE', #1092, #3840 ) ;
#7138=EDGE_CURVE ( 'NONE', #4408, #8429, #1044, .T. ) ;
#7143=CYLINDRICAL_SURFACE ( 'NONE', #6640, 1.000000000000000888 ) ;
#7145=CARTESIAN_POINT ( 'NONE',  ( -35.35889894354067309, -7.999999999999996447, -25.00000000000000000 ) ) ;
#7148=EDGE_CURVE ( 'NONE', #1046, #2177, #3160, .T. ) ;
#7155=EDGE_CURVE ( 'NONE', #5681, #772, #7521, .T. ) ;
#7163=EDGE_CURVE ( 'NONE', #3431, #7971, #2034, .T. ) ;
#7176=ORIENTED_EDGE ( 'NONE', *, *, #4128, .T. ) ;
#7178=ADVANCED_FACE ( 'NONE', ( #6988 ), #3647, .F. ) ;
#7181=ORIENTED_EDGE ( 'NONE', *, *, #1157, .F. ) ;
#7184=DIRECTION ( 'NONE',  ( -1.000000000000000000, 0.000000000000000000, 0.000000000000000000 ) ) ;
#7186=AXIS2_PLACEMENT_3D ( 'NONE', #3669, #5073, #3096 ) ;
#7211=EDGE_LOOP ( 'NONE', ( #4212, #7718, #5730, #733 ) ) ;
#7232=LINE ( 'NONE', #1235, #5444 ) ;
#7239=ADVANCED_FACE ( 'NONE', ( #1793 ), #7784, .T. ) ;
#7248=CARTESIAN_POINT ( 'NONE',  ( -17.99999999999998579, 1.469576158976828483E-15, -26.00000000000000355 ) ) ;
#7256=LINE ( 'NONE', #2425, #7641 ) ;
#7260=ORIENTED_EDGE ( 'NONE', *, *, #2646, .T. ) ;
#7263=AXIS2_PLACEMENT_3D ( 'NONE', #2322, #7184, #8358 ) ;
#7275=DIRECTION ( 'NONE',  ( -0.000000000000000000, -1.000000000000000000, 0.000000000000000000 ) ) ;
#7284=CARTESIAN_POINT ( 'NONE',  ( -18.00000000000002132, 1.469576158976823947E-15, -29.65000000000000213 ) ) ;
#7288=CARTESIAN_POINT ( 'NONE',  ( -41.99999999999981526, 0.000000000000000000, -45.00000000000000000 ) ) ;
#7292=ORIENTED_EDGE ( 'NONE', *, *, #5691, .F. ) ;
#7293=DIRECTION ( 'NONE',  ( 0.000000000000000000, 1.000000000000000000, -0.000000000000000000 ) ) ;
#7304=ADVANCED_FACE ( 'NONE', ( #8370 ), #331, .T. ) ;
#7308=DIRECTION ( 'NONE',  ( -1.000000000000000000, 0.000000000000000000, 0.000000000000000000 ) ) ;
#7328=AXIS2_PLACEMENT_3D ( 'NONE', #469, #4585, #3882 ) ;
#7331=DIRECTION ( 'NONE',  ( 0.000000000000000000, 0.000000000000000000, 1.000000000000000000 ) ) ;
#7332=EDGE_CURVE ( 'NONE', #6167, #7794, #3119, .T. ) ;
#7336=DIRECTION ( 'NONE',  ( 0.000000000000000000, 0.000000000000000000, 1.000000000000000000 ) ) ;
#7340=MECHANICAL_DESIGN_GEOMETRIC_PRESENTATION_REPRESENTATION('',(#2427),#5791);
#7360=AXIS2_PLACEMENT_3D ( 'NONE', #1590, #6920, #5032 ) ;
#7361=VECTOR ( 'NONE', #5061, 1000.000000000000000 ) ;
#7363=AXIS2_PLACEMENT_3D ( 'NONE', #2674, #16, #8096 ) ;
#7366=CARTESIAN_POINT ( 'NONE',  ( -40.00000000000002842, 1.224646799147353059E-15, -41.34999999999999432 ) ) ;
#7374=EDGE_CURVE ( 'NONE', #3127, #8141, #2671, .T. ) ;
#7380=DIRECTION ( 'NONE',  ( 0.000000000000000000, 0.000000000000000000, -1.000000000000000000 ) ) ;
#7390=PRESENTATION_STYLE_ASSIGNMENT (( #6631 ) ) ;
#7409=CARTESIAN_POINT ( 'NONE',  ( -30.00000000000002842, 0.000000000000000000, -44.00000000000000000 ) ) ;
#7411=EDGE_CURVE ( 'NONE', #3121, #3466, #6258, .T. ) ;
#7417=AXIS2_PLACEMENT_3D ( 'NONE', #2945, #4792, #2155 ) ;
#7423=DIRECTION ( 'NONE',  ( 1.000000000000000000, 0.000000000000000000, 0.000000000000000000 ) ) ;
#7425=ORIENTED_EDGE ( 'NONE', *, *, #7917, .T. ) ;
#7437=DIRECTION ( 'NONE',  ( 0.000000000000000000, -1.000000000000000000, 0.000000000000000000 ) ) ;
#7439=ORIENTED_EDGE ( 'NONE', *, *, #4150, .T. ) ;
#7448=EDGE_CURVE ( 'NONE', #772, #8337, #4516, .T. ) ;
#7472=VERTEX_POINT ( 'NONE', #487 ) ;
#7478=CARTESIAN_POINT ( 'NONE',  ( -25.64110105645932336, -8.999999999999998224, 124.0000000000000000 ) ) ;
#7490=AXIS2_PLACEMENT_3D ( 'NONE', #460, #8583, #5852 ) ;
#7492=CARTESIAN_POINT ( 'NONE',  ( -26.64110105645932336, 10.00000000000000178, -24.00000000000000000 ) ) ;
#7494=AXIS2_PLACEMENT_3D ( 'NONE', #5767, #5023, #1719 ) ;
#7506=CARTESIAN_POINT ( 'NONE',  ( -34.35889894354067309, 8.000000000000000000, 125.0000000000000000 ) ) ;
#7507=DIRECTION ( 'NONE',  ( -1.000000000000000000, 0.000000000000000000, -0.000000000000000000 ) ) ;
#7511=EDGE_LOOP ( 'NONE', ( #7181, #8095 ) ) ;
#7521=LINE ( 'NONE', #1481, #2175 ) ;
#7523=ORIENTED_EDGE ( 'NONE', *, *, #8138, .F. ) ;
#7524=EDGE_CURVE ( 'NONE', #2150, #1009, #8509, .T. ) ;
#7529=CYLINDRICAL_SURFACE ( 'NONE', #627, 10.00000000000000178 ) ;
#7531=DIRECTION ( 'NONE',  ( 1.000000000000000000, 0.000000000000000000, 0.000000000000000000 ) ) ;
#7551=CARTESIAN_POINT ( 'NONE',  ( -26.64110105645932336, 8.000000000000000000, -23.99999999999999289 ) ) ;
#7565=VECTOR ( 'NONE', #1905, 1000.000000000000000 ) ;
#7572=ADVANCED_FACE ( 'NONE', ( #2626 ), #1332, .T. ) ;
#7591=DIRECTION ( 'NONE',  ( -0.000000000000000000, -0.000000000000000000, -1.000000000000000000 ) ) ;
#7592=DIRECTION ( 'NONE',  ( 0.000000000000000000, 0.000000000000000000, 1.000000000000000000 ) ) ;
#7594=FACE_BOUND ( 'NONE', #4581, .T. ) ;
#7595=ORIENTED_EDGE ( 'NONE', *, *, #5163, .F. ) ;
#7602=DIRECTION ( 'NONE',  ( -0.000000000000000000, 0.000000000000000000, -1.000000000000000000 ) ) ;
#7603=CIRCLE ( 'NONE', #3247, 11.99999999999983302 ) ;
#7606=DIRECTION ( 'NONE',  ( 1.000000000000000000, 0.000000000000000000, -0.000000000000000000 ) ) ;
#7609=VERTEX_POINT ( 'NONE', #2537 ) ;
#7613=ORIENTED_EDGE ( 'NONE', *, *, #2526, .F. ) ;
#7623=DIRECTION ( 'NONE',  ( 1.000000000000000000, 0.000000000000000000, -0.000000000000000000 ) ) ;
#7630=AXIS2_PLACEMENT_3D ( 'NONE', #3789, #8383, #342 ) ;
#7638=EDGE_LOOP ( 'NONE', ( #955, #661, #4844, #8101 ) ) ;
#7641=VECTOR ( 'NONE', #5935, 1000.000000000000000 ) ;
#7645=EDGE_CURVE ( 'NONE', #7609, #1046, #1287, .T. ) ;
#7649=CARTESIAN_POINT ( 'NONE',  ( -34.35889894354067309, -8.999999999999998224, 124.0000000000000000 ) ) ;
#7656=VECTOR ( 'NONE', #7437, 1000.000000000000000 ) ;
#7664=DIRECTION ( 'NONE',  ( 0.000000000000000000, 0.000000000000000000, 1.000000000000000000 ) ) ;
#7681=ADVANCED_FACE ( 'NONE', ( #8042 ), #2003, .F. ) ;
#7682=DIRECTION ( 'NONE',  ( 0.000000000000000000, 0.000000000000000000, -1.000000000000000000 ) ) ;
#7687=CARTESIAN_POINT ( 'NONE',  ( -35.35889894354067309, 8.000000000000000000, -25.00000000000000000 ) ) ;
#7690=AXIS2_PLACEMENT_3D ( 'NONE', #2967, #1679, #4943 ) ;
#7693=AXIS2_PLACEMENT_3D ( 'NONE', #8142, #2101, #4784 ) ;
#7702=EDGE_CURVE ( 'NONE', #3069, #6952, #2601, .T. ) ;
#7718=ORIENTED_EDGE ( 'NONE', *, *, #2699, .T. ) ;
#7744=AXIS2_PLACEMENT_3D ( 'NONE', #4908, #2757, #806 ) ;
#7756=ORIENTED_EDGE ( 'NONE', *, *, #886, .T. ) ;
#7759=VECTOR ( 'NONE', #5757, 1000.000000000000000 ) ;
#7764=CARTESIAN_POINT ( 'NONE',  ( -34.35889894354067309, -8.999999999999998224, 125.0000000000000000 ) ) ;
#7767=DIRECTION ( 'NONE',  ( -0.000000000000000000, -0.000000000000000000, -1.000000000000000000 ) ) ;
#7777=CIRCLE ( 'NONE', #6925, 12.00000000000000000 ) ;
#7784=CYLINDRICAL_SURFACE ( 'NONE', #4279, 10.00000000000000178 ) ;
#7787=CARTESIAN_POINT ( 'NONE',  ( 0.000000000000000000, 0.000000000000000000, 0.000000000000000000 ) ) ;
#7788=ORIENTED_EDGE ( 'NONE', *, *, #5099, .F. ) ;
#7794=VERTEX_POINT ( 'NONE', #5165 ) ;
#7797=DIRECTION ( 'NONE',  ( 0.000000000000000000, 0.000000000000000000, -1.000000000000000000 ) ) ;
#7799=CARTESIAN_POINT ( 'NONE',  ( -30.00000000000002842, 0.000000000000000000, -28.65000000000000213 ) ) ;
#7823=CIRCLE ( 'NONE', #1776, 11.99999999999979217 ) ;
#7825=PLANE ( 'NONE',  #6851 ) ;
#7838=CARTESIAN_POINT ( 'NONE',  ( -25.64110105645932336, -8.999999999999998224, 125.0000000000000000 ) ) ;
#7842=ORIENTED_EDGE ( 'NONE', *, *, #6341, .F. ) ;
#7846=EDGE_LOOP ( 'NONE', ( #6377, #4654, #6684, #1583 ) ) ;
#7854=DIRECTION ( 'NONE',  ( -0.000000000000000000, 0.000000000000000000, -1.000000000000000000 ) ) ;
#7866=CARTESIAN_POINT ( 'NONE',  ( -30.00000000000002842, 0.000000000000000000, -29.65000000000000213 ) ) ;
#7880=EDGE_CURVE ( 'NONE', #8429, #4408, #4268, .T. ) ;
#7886=ORIENTED_EDGE ( 'NONE', *, *, #8086, .T. ) ;
#7893=ADVANCED_FACE ( 'NONE', ( #4904 ), #8079, .F. ) ;
#7897=DIRECTION ( 'NONE',  ( -0.000000000000000000, -0.000000000000000000, -1.000000000000000000 ) ) ;
#7901=ORIENTED_EDGE ( 'NONE', *, *, #7524, .F. ) ;
#7906=FACE_BOUND ( 'NONE', #959, .T. ) ;
#7907=DIRECTION ( 'NONE',  ( -1.000000000000000000, 0.000000000000000000, 0.000000000000000000 ) ) ;
#7914=AXIS2_PLACEMENT_3D ( 'NONE', #5635, #7664, #2300 ) ;
#7917=EDGE_CURVE ( 'NONE', #1009, #5895, #5372, .T. ) ;
#7925=DIRECTION ( 'NONE',  ( 0.000000000000000000, 0.000000000000000000, 1.000000000000000000 ) ) ;
#7937=ADVANCED_FACE ( 'NONE', ( #6700 ), #4195, .T. ) ;
#7941=EDGE_CURVE ( 'NONE', #8141, #5715, #52, .T. ) ;
#7944=VERTEX_POINT ( 'NONE', #5461 ) ;
#7954=DIRECTION ( 'NONE',  ( 1.000000000000000000, -0.000000000000000000, -0.000000000000000000 ) ) ;
#7957=ORIENTED_EDGE ( 'NONE', *, *, #4150, .F. ) ;
#7963=ORIENTED_EDGE ( 'NONE', *, *, #1148, .F. ) ;
#7967=CARTESIAN_POINT ( 'NONE',  ( -18.00000000000002132, 1.469576158976823947E-15, -28.65000000000000213 ) ) ;
#7971=VERTEX_POINT ( 'NONE', #6831 ) ;
#7981=AXIS2_PLACEMENT_3D ( 'NONE', #1395, #731, #6162 ) ;
#7988=CARTESIAN_POINT ( 'NONE',  ( -35.35889894354067309, -7.999999999999996447, -24.00000000000000000 ) ) ;
#8001=DIRECTION ( 'NONE',  ( 0.000000000000000000, 1.000000000000000000, 0.000000000000000000 ) ) ;
#8016=ORIENTED_EDGE ( 'NONE', *, *, #7645, .F. ) ;
#8019=EDGE_LOOP ( 'NONE', ( #6373, #2804, #1994, #2433 ) ) ;
#8025=DIRECTION ( 'NONE',  ( -1.000000000000000000, 0.000000000000000000, 0.000000000000000000 ) ) ;
#8042=FACE_OUTER_BOUND ( 'NONE', #8019, .T. ) ;
#8044=( LENGTH_UNIT ( ) NAMED_UNIT ( * ) SI_UNIT ( .MILLI., .METRE. ) );
#8051=ORIENTED_EDGE ( 'NONE', *, *, #7702, .F. ) ;
#8060=ADVANCED_FACE ( 'NONE', ( #6220 ), #4153, .T. ) ;
#8062=AXIS2_PLACEMENT_3D ( 'NONE', #7764, #1732, #4418 ) ;
#8071=COLOUR_RGB ( '', 0.31764706, 0.68627451, 0.89019608) ;
#8073=ADVANCED_FACE ( 'NONE', ( #4862 ), #5554, .T. ) ;
#8077=EDGE_CURVE ( 'NONE', #7944, #7472, #4372, .T. ) ;
#8079=CYLINDRICAL_SURFACE ( 'NONE', #3839, 1.000000000000000888 ) ;
#8080=AXIS2_PLACEMENT_3D ( 'NONE', #5887, #2497, #8660 ) ;
#8086=EDGE_CURVE ( 'NONE', #3680, #7609, #2307, .T. ) ;
#8091=DIRECTION ( 'NONE',  ( 1.000000000000000000, 0.000000000000000000, 0.000000000000000000 ) ) ;
#8094=SHAPE_REPRESENTATION_RELATIONSHIP ( 'NONE' , 'NONE' ,  #4062, #2772 ) ;
#8095=ORIENTED_EDGE ( 'NONE', *, *, #6769, .F. ) ;
#8096=DIRECTION ( 'NONE',  ( 1.000000000000000000, 0.000000000000000000, 0.000000000000000000 ) ) ;
#8100=EDGE_CURVE ( 'NONE', #1663, #5109, #3569, .T. ) ;
#8101=ORIENTED_EDGE ( 'NONE', *, *, #8303, .F. ) ;
#8108=DIRECTION ( 'NONE',  ( 1.000000000000000000, 0.000000000000000000, -0.000000000000000000 ) ) ;
#8109=ORIENTED_EDGE ( 'NONE', *, *, #4546, .F. ) ;
#8112=AXIS2_PLACEMENT_3D ( 'NONE', #8437, #5649, #6399 ) ;
#8133=CIRCLE ( 'NONE', #653, 1.000000000000000888 ) ;
#8138=EDGE_CURVE ( 'NONE', #3221, #2177, #224, .T. ) ;
#8141=VERTEX_POINT ( 'NONE', #931 ) ;
#8142=CARTESIAN_POINT ( 'NONE',  ( -33.35889894354067309, 8.000000000000000000, -23.99999999999999289 ) ) ;
#8155=DIRECTION ( 'NONE',  ( 0.000000000000000000, 1.000000000000000000, 0.000000000000000000 ) ) ;
#8171=DIRECTION ( 'NONE',  ( -1.000000000000000000, 0.000000000000000000, 0.000000000000000000 ) ) ;
#8180=EDGE_CURVE ( 'NONE', #772, #1675, #1982, .T. ) ;
#8182=CARTESIAN_POINT ( 'NONE',  ( -33.35889894354067309, 8.000000000000000000, -23.99999999999999289 ) ) ;
#8186=EDGE_LOOP ( 'NONE', ( #8690, #7788, #5718, #3468 ) ) ;
#8190=CIRCLE ( 'NONE', #706, 1.000000000000000888 ) ;
#8213=AXIS2_PLACEMENT_3D ( 'NONE', #2918, #8252, #4982 ) ;
#8228=ORIENTED_EDGE ( 'NONE', *, *, #7448, .T. ) ;
#8236=EDGE_LOOP ( 'NONE', ( #3597, #3342, #3723, #2367 ) ) ;
#8239=CYLINDRICAL_SURFACE ( 'NONE', #5162, 1.000000000000000888 ) ;
#8252=DIRECTION ( 'NONE',  ( -0.000000000000000000, -0.000000000000000000, -1.000000000000000000 ) ) ;
#8254=EDGE_CURVE ( 'NONE', #2617, #3764, #2352, .T. ) ;
#8266=PLANE ( 'NONE',  #7744 ) ;
#8270=EDGE_LOOP ( 'NONE', ( #2811, #2937, #8626, #7260 ) ) ;
#8282=FACE_OUTER_BOUND ( 'NONE', #6744, .T. ) ;
#8285=FACE_OUTER_BOUND ( 'NONE', #4926, .T. ) ;
#8297=ORIENTED_EDGE ( 'NONE', *, *, #771, .T. ) ;
#8303=EDGE_CURVE ( 'NONE', #5475, #5184, #1681, .T. ) ;
#8305=CARTESIAN_POINT ( 'NONE',  ( -30.00000000000002487, 0.000000000000000000, -29.65000000000000213 ) ) ;
#8322=DIRECTION ( 'NONE',  ( -1.000000000000000000, 0.000000000000000000, 0.000000000000000000 ) ) ;
#8325=DIRECTION ( 'NONE',  ( 0.000000000000000000, 0.000000000000000000, 1.000000000000000000 ) ) ;
#8337=VERTEX_POINT ( 'NONE', #6307 ) ;
#8345=DIRECTION ( 'NONE',  ( 1.000000000000000000, 0.000000000000000000, 0.000000000000000000 ) ) ;
#8346=EDGE_CURVE ( 'NONE', #7944, #4956, #157, .T. ) ;
#8352=DIRECTION ( 'NONE',  ( 0.000000000000000000, 0.000000000000000000, 1.000000000000000000 ) ) ;
#8358=DIRECTION ( 'NONE',  ( 0.000000000000000000, 0.000000000000000000, 1.000000000000000000 ) ) ;
#8370=FACE_OUTER_BOUND ( 'NONE', #3578, .T. ) ;
#8377=ADVANCED_FACE ( 'NONE', ( #1731, #4416 ), #390, .F. ) ;
#8378=EDGE_LOOP ( 'NONE', ( #1254, #1801, #1604, #1558 ) ) ;
#8383=DIRECTION ( 'NONE',  ( -0.000000000000000000, -0.000000000000000000, -1.000000000000000000 ) ) ;
#8407=CIRCLE ( 'NONE', #2779, 1.000000000000000888 ) ;
#8409=DIRECTION ( 'NONE',  ( -0.000000000000000000, -0.000000000000000000, -1.000000000000000000 ) ) ;
#8427=ORIENTED_EDGE ( 'NONE', *, *, #6921, .T. ) ;
#8429=VERTEX_POINT ( 'NONE', #1901 ) ;
#8437=CARTESIAN_POINT ( 'NONE',  ( -26.64110105645932336, -7.999999999999996447, -23.99999999999999289 ) ) ;
#8442=EDGE_CURVE ( 'NONE', #598, #5405, #3115, .T. ) ;
#8454=AXIS2_PLACEMENT_3D ( 'NONE', #5651, #7014, #8352 ) ;
#8463=FACE_OUTER_BOUND ( 'NONE', #7211, .T. ) ;
#8465=DIRECTION ( 'NONE',  ( 0.000000000000000000, 0.000000000000000000, -1.000000000000000000 ) ) ;
#8473=CARTESIAN_POINT ( 'NONE',  ( -30.00000000000019185, 0.000000000000000000, -41.34999999999999432 ) ) ;
#8479=CARTESIAN_POINT ( 'NONE',  ( -33.35889894354067309, 10.00000000000000178, -24.00000000000000000 ) ) ;
#8487=CARTESIAN_POINT ( 'NONE',  ( -26.64110105645932336, -8.999999999999998224, 124.0000000000000000 ) ) ;
#8491=AXIS2_PLACEMENT_3D ( 'NONE', #7838, #5106, #7797 ) ;
#8495=CARTESIAN_POINT ( 'NONE',  ( -25.64110105645932336, -7.999999999999996447, 124.0000000000000000 ) ) ;
#8499=CIRCLE ( 'NONE', #5822, 2.000000000000001776 ) ;
#8503=DIRECTION ( 'NONE',  ( -1.000000000000000000, 0.000000000000000000, 0.000000000000000000 ) ) ;
#8504=DIRECTION ( 'NONE',  ( -0.000000000000000000, 1.000000000000000000, -0.000000000000000000 ) ) ;
#8509=CIRCLE ( 'NONE', #8080, 11.99999999999983302 ) ;
#8511=EDGE_CURVE ( 'NONE', #1675, #7794, #8190, .T. ) ;
#8514=DIRECTION ( 'NONE',  ( -0.000000000000000000, -0.000000000000000000, -1.000000000000000000 ) ) ;
#8515=CARTESIAN_POINT ( 'NONE',  ( -34.35889894354067309, -7.999999999999996447, 124.0000000000000000 ) ) ;
#8518=CARTESIAN_POINT ( 'NONE',  ( -20.00000000000002487, 0.000000000000000000, -29.65000000000000213 ) ) ;
#8524=EDGE_CURVE ( 'NONE', #3779, #6167, #5366, .T. ) ;
#8526=DIRECTION ( 'NONE',  ( 1.000000000000000000, 0.000000000000000000, 0.000000000000000000 ) ) ;
#8530=DIRECTION ( 'NONE',  ( 0.000000000000000000, 0.000000000000000000, -1.000000000000000000 ) ) ;
#8532=AXIS2_PLACEMENT_3D ( 'NONE', #7008, #7623, #4281 ) ;
#8535=CARTESIAN_POINT ( 'NONE',  ( -40.00000000000002842, 1.224646799147353059E-15, -28.65000000000000213 ) ) ;
#8544=EDGE_CURVE ( 'NONE', #6933, #1925, #849, .T. ) ;
#8545=CARTESIAN_POINT ( 'NONE',  ( -30.00000000000002487, 0.000000000000000000, -29.65000000000000213 ) ) ;
#8549=VECTOR ( 'NONE', #6443, 1000.000000000000000 ) ;
#8551=VERTEX_POINT ( 'NONE', #4970 ) ;
#8557=FACE_OUTER_BOUND ( 'NONE', #6907, .T. ) ;
#8558=CIRCLE ( 'NONE', #4058, 1.000000000000000888 ) ;
#8559=CARTESIAN_POINT ( 'NONE',  ( -25.64110105645932336, 8.000000000000000000, -24.00000000000000000 ) ) ;
#8564=ORIENTED_EDGE ( 'NONE', *, *, #4199, .T. ) ;
#8569=FACE_OUTER_BOUND ( 'NONE', #2869, .T. ) ;
#8575=FILL_AREA_STYLE_COLOUR ( '', #6214 ) ;
#8576=ORIENTED_EDGE ( 'NONE', *, *, #4546, .T. ) ;
#8583=DIRECTION ( 'NONE',  ( -0.000000000000000000, -0.000000000000000000, -1.000000000000000000 ) ) ;
#8589=EDGE_CURVE ( 'NONE', #5405, #8551, #998, .T. ) ;
#8592=ORIENTED_EDGE ( 'NONE', *, *, #1148, .T. ) ;
#8616=VECTOR ( 'NONE', #2018, 1000.000000000000000 ) ;
#8618=CARTESIAN_POINT ( 'NONE',  ( -33.35889894354067309, 8.000000000000000000, 125.0000000000000000 ) ) ;
#8626=ORIENTED_EDGE ( 'NONE', *, *, #2573, .T. ) ;
#8627=AXIS2_PLACEMENT_3D ( 'NONE', #862, #3604, #5489 ) ;
#8629=LINE ( 'NONE', #1805, #5112 ) ;
#8645=AXIS2_PLACEMENT_3D ( 'NONE', #8182, #7592, #5562 ) ;
#8649=EDGE_CURVE ( 'NONE', #1675, #7609, #3492, .T. ) ;
#8659=SPHERICAL_SURFACE ( 'NONE', #1978, 1.000000000000000000 ) ;
#8660=DIRECTION ( 'NONE',  ( -1.000000000000000000, 0.000000000000000000, 0.000000000000000000 ) ) ;
#8663=CARTESIAN_POINT ( 'NONE',  ( -26.64110105645932336, 8.000000000000000000, 124.0000000000000000 ) ) ;
#8687=DIRECTION ( 'NONE',  ( -1.000000000000000000, 0.000000000000000000, 0.000000000000000000 ) ) ;
#8690=ORIENTED_EDGE ( 'NONE', *, *, #5229, .F. ) ;
#8695=CARTESIAN_POINT ( 'NONE',  ( -33.35889894354067309, 8.000000000000000000, 124.0000000000000000 ) ) ;
#8707=ORIENTED_EDGE ( 'NONE', *, *, #3311, .F. ) ;
#8708=ORIENTED_EDGE ( 'NONE', *, *, #1464, .T. ) ;
#8713=CARTESIAN_POINT ( 'NONE',  ( -40.00000000000002842, 1.224646799147353059E-15, -44.00000000000000000 ) ) ;
#8715=ORIENTED_EDGE ( 'NONE', *, *, #5502, .T. ) ;
#8717=DIRECTION ( 'NONE',  ( -1.000000000000000000, 0.000000000000000000, 0.000000000000000000 ) ) ;
ENDSEC;
END-ISO-10303-21;
